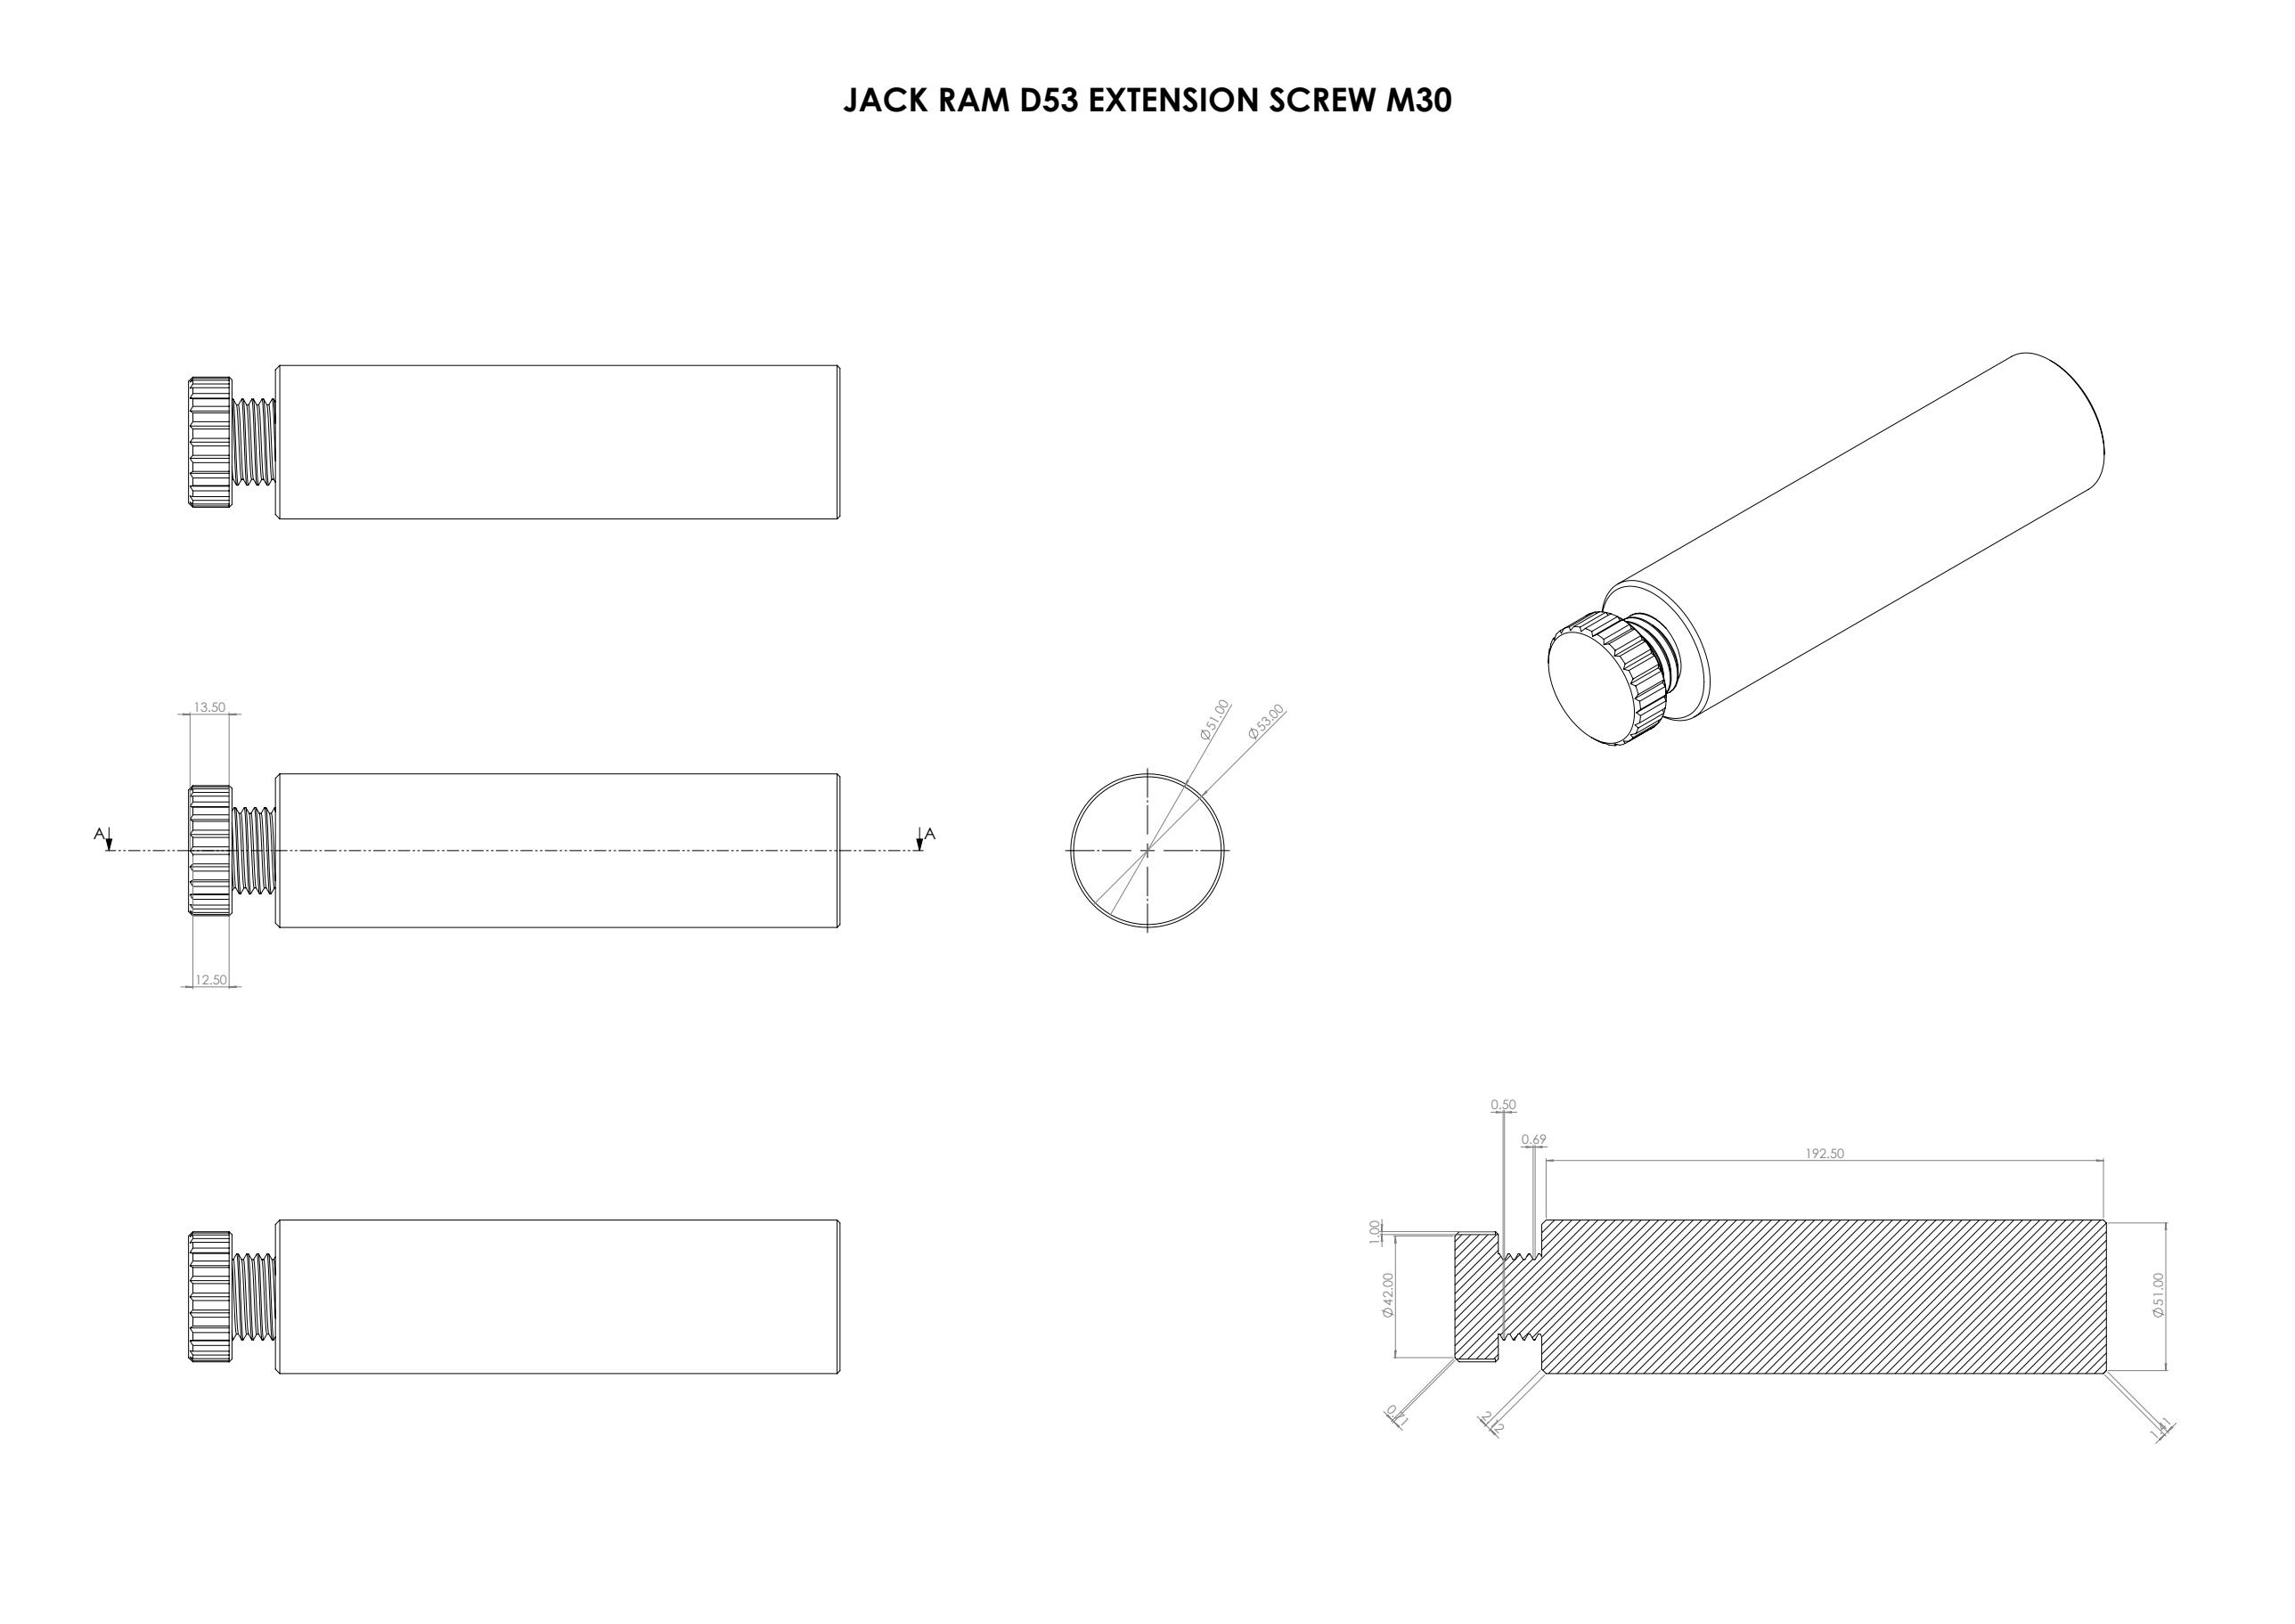
ISO-10303-21;
HEADER;
/* Generated by software containing ST-Developer
 * from STEP Tools, Inc. (www.steptools.com) 
 */

FILE_DESCRIPTION(
/* description */ (''),
/* implementation_level */ '2;1');

FILE_NAME(
/* name */ '10_Jack_Ram_D53_Extension_Screw_M30.step',
/* time_stamp */ '2026-10-20T10:03:03-07:00',
/* author */ (''),
/* organization */ (''),
/* preprocessor_version */ 'ST-DEVELOPER v20.2',
/* originating_system */ 'Autodesk Translation Framework v15.15.0.0',
/* authorisation */ '');

FILE_SCHEMA (('AUTOMOTIVE_DESIGN { 1 0 10303 214 3 1 1 }'));
ENDSEC;

DATA;
#10=MECHANICAL_DESIGN_GEOMETRIC_PRESENTATION_REPRESENTATION('',(#529),#71492);
#271=(
BOUNDED_CURVE()
B_SPLINE_CURVE(2,(#44561,#44562,#44563),.UNSPECIFIED.,.F.,.F.)
B_SPLINE_CURVE_WITH_KNOTS((3,3),(0.,0.186897942309885),.UNSPECIFIED.)
CURVE()
GEOMETRIC_REPRESENTATION_ITEM()
RATIONAL_B_SPLINE_CURVE((1.,1.00104922243968,1.00074449035823))
REPRESENTATION_ITEM('')
);
#272=(
BOUNDED_CURVE()
B_SPLINE_CURVE(2,(#44566,#44567,#44568),.UNSPECIFIED.,.F.,.F.)
B_SPLINE_CURVE_WITH_KNOTS((3,3),(0.102768382432289,0.289666324741965),
 .UNSPECIFIED.)
CURVE()
GEOMETRIC_REPRESENTATION_ITEM()
RATIONAL_B_SPLINE_CURVE((1.00074449035274,1.00104922243194,1.))
REPRESENTATION_ITEM('')
);
#273=(
BOUNDED_CURVE()
B_SPLINE_CURVE(2,(#44582,#44583,#44584),.UNSPECIFIED.,.F.,.F.)
B_SPLINE_CURVE_WITH_KNOTS((3,3),(0.,0.186897942309674),.UNSPECIFIED.)
CURVE()
GEOMETRIC_REPRESENTATION_ITEM()
RATIONAL_B_SPLINE_CURVE((1.,1.00104922243196,1.00074449035276))
REPRESENTATION_ITEM('')
);
#274=(
BOUNDED_CURVE()
B_SPLINE_CURVE(2,(#44587,#44588,#44589),.UNSPECIFIED.,.F.,.F.)
B_SPLINE_CURVE_WITH_KNOTS((3,3),(0.102768382432294,0.289666324741965),
 .UNSPECIFIED.)
CURVE()
GEOMETRIC_REPRESENTATION_ITEM()
RATIONAL_B_SPLINE_CURVE((1.00074449035267,1.00104922243184,1.))
REPRESENTATION_ITEM('')
);
#275=(
BOUNDED_CURVE()
B_SPLINE_CURVE(2,(#44603,#44604,#44605),.UNSPECIFIED.,.F.,.F.)
B_SPLINE_CURVE_WITH_KNOTS((3,3),(0.,0.186897942309901),.UNSPECIFIED.)
CURVE()
GEOMETRIC_REPRESENTATION_ITEM()
RATIONAL_B_SPLINE_CURVE((1.,1.00104922243998,1.00074449035845))
REPRESENTATION_ITEM('')
);
#276=(
BOUNDED_CURVE()
B_SPLINE_CURVE(2,(#44608,#44609,#44610),.UNSPECIFIED.,.F.,.F.)
B_SPLINE_CURVE_WITH_KNOTS((3,3),(0.102768382432298,0.289666324741965),
 .UNSPECIFIED.)
CURVE()
GEOMETRIC_REPRESENTATION_ITEM()
RATIONAL_B_SPLINE_CURVE((1.00074449035256,1.00104922243169,1.))
REPRESENTATION_ITEM('')
);
#277=(
BOUNDED_CURVE()
B_SPLINE_CURVE(2,(#44624,#44625,#44626),.UNSPECIFIED.,.F.,.F.)
B_SPLINE_CURVE_WITH_KNOTS((3,3),(0.,0.186897942309885),.UNSPECIFIED.)
CURVE()
GEOMETRIC_REPRESENTATION_ITEM()
RATIONAL_B_SPLINE_CURVE((1.,1.00104922243968,1.00074449035823))
REPRESENTATION_ITEM('')
);
#278=(
BOUNDED_CURVE()
B_SPLINE_CURVE(2,(#44629,#44630,#44631),.UNSPECIFIED.,.F.,.F.)
B_SPLINE_CURVE_WITH_KNOTS((3,3),(0.102768382432289,0.289666324741965),
 .UNSPECIFIED.)
CURVE()
GEOMETRIC_REPRESENTATION_ITEM()
RATIONAL_B_SPLINE_CURVE((1.00074449035274,1.00104922243194,1.))
REPRESENTATION_ITEM('')
);
#279=(
BOUNDED_CURVE()
B_SPLINE_CURVE(2,(#44645,#44646,#44647),.UNSPECIFIED.,.F.,.F.)
B_SPLINE_CURVE_WITH_KNOTS((3,3),(0.,0.186897942309671),.UNSPECIFIED.)
CURVE()
GEOMETRIC_REPRESENTATION_ITEM()
RATIONAL_B_SPLINE_CURVE((1.,1.00104922243187,1.00074449035269))
REPRESENTATION_ITEM('')
);
#280=(
BOUNDED_CURVE()
B_SPLINE_CURVE(2,(#44650,#44651,#44652),.UNSPECIFIED.,.F.,.F.)
B_SPLINE_CURVE_WITH_KNOTS((3,3),(0.102768382432295,0.289666324741964),
 .UNSPECIFIED.)
CURVE()
GEOMETRIC_REPRESENTATION_ITEM()
RATIONAL_B_SPLINE_CURVE((1.00074449035266,1.00104922243182,1.))
REPRESENTATION_ITEM('')
);
#281=(
BOUNDED_CURVE()
B_SPLINE_CURVE(2,(#44666,#44667,#44668),.UNSPECIFIED.,.F.,.F.)
B_SPLINE_CURVE_WITH_KNOTS((3,3),(0.,0.186897942309672),.UNSPECIFIED.)
CURVE()
GEOMETRIC_REPRESENTATION_ITEM()
RATIONAL_B_SPLINE_CURVE((1.,1.00104922243174,1.0007444903526))
REPRESENTATION_ITEM('')
);
#282=(
BOUNDED_CURVE()
B_SPLINE_CURVE(2,(#44671,#44672,#44673),.UNSPECIFIED.,.F.,.F.)
B_SPLINE_CURVE_WITH_KNOTS((3,3),(0.102768382432307,0.289666324741965),
 .UNSPECIFIED.)
CURVE()
GEOMETRIC_REPRESENTATION_ITEM()
RATIONAL_B_SPLINE_CURVE((1.00074449035222,1.00104922243121,1.))
REPRESENTATION_ITEM('')
);
#283=(
BOUNDED_CURVE()
B_SPLINE_CURVE(2,(#44689,#44690,#44691),.UNSPECIFIED.,.F.,.F.)
B_SPLINE_CURVE_WITH_KNOTS((3,3),(0.,0.186897942309665),.UNSPECIFIED.)
CURVE()
GEOMETRIC_REPRESENTATION_ITEM()
RATIONAL_B_SPLINE_CURVE((1.,1.00104922243153,1.00074449035245))
REPRESENTATION_ITEM('')
);
#284=(
BOUNDED_CURVE()
B_SPLINE_CURVE(2,(#44694,#44695,#44696),.UNSPECIFIED.,.F.,.F.)
B_SPLINE_CURVE_WITH_KNOTS((3,3),(0.102768382432301,0.289666324741966),
 .UNSPECIFIED.)
CURVE()
GEOMETRIC_REPRESENTATION_ITEM()
RATIONAL_B_SPLINE_CURVE((1.00074449035228,1.00104922243129,1.))
REPRESENTATION_ITEM('')
);
#285=(
BOUNDED_CURVE()
B_SPLINE_CURVE(2,(#44710,#44711,#44712),.UNSPECIFIED.,.F.,.F.)
B_SPLINE_CURVE_WITH_KNOTS((3,3),(0.,0.18689794230967),.UNSPECIFIED.)
CURVE()
GEOMETRIC_REPRESENTATION_ITEM()
RATIONAL_B_SPLINE_CURVE((1.,1.00104922243168,1.00074449035256))
REPRESENTATION_ITEM('')
);
#286=(
BOUNDED_CURVE()
B_SPLINE_CURVE(2,(#44715,#44716,#44717),.UNSPECIFIED.,.F.,.F.)
B_SPLINE_CURVE_WITH_KNOTS((3,3),(0.10276838243214,0.289666324741965),
 .UNSPECIFIED.)
CURVE()
GEOMETRIC_REPRESENTATION_ITEM()
RATIONAL_B_SPLINE_CURVE((1.00074449035625,1.00104922243688,1.))
REPRESENTATION_ITEM('')
);
#287=(
BOUNDED_CURVE()
B_SPLINE_CURVE(2,(#44731,#44732,#44733),.UNSPECIFIED.,.F.,.F.)
B_SPLINE_CURVE_WITH_KNOTS((3,3),(0.,0.186897942309663),.UNSPECIFIED.)
CURVE()
GEOMETRIC_REPRESENTATION_ITEM()
RATIONAL_B_SPLINE_CURVE((1.,1.00104922243133,1.00074449035231))
REPRESENTATION_ITEM('')
);
#288=(
BOUNDED_CURVE()
B_SPLINE_CURVE(2,(#44736,#44737,#44738),.UNSPECIFIED.,.F.,.F.)
B_SPLINE_CURVE_WITH_KNOTS((3,3),(0.102768382432299,0.289666324741965),
 .UNSPECIFIED.)
CURVE()
GEOMETRIC_REPRESENTATION_ITEM()
RATIONAL_B_SPLINE_CURVE((1.00074449035251,1.00104922243162,1.))
REPRESENTATION_ITEM('')
);
#289=(
BOUNDED_CURVE()
B_SPLINE_CURVE(2,(#44752,#44753,#44754),.UNSPECIFIED.,.F.,.F.)
B_SPLINE_CURVE_WITH_KNOTS((3,3),(0.,0.186897942309671),.UNSPECIFIED.)
CURVE()
GEOMETRIC_REPRESENTATION_ITEM()
RATIONAL_B_SPLINE_CURVE((1.,1.00104922243163,1.00074449035252))
REPRESENTATION_ITEM('')
);
#290=(
BOUNDED_CURVE()
B_SPLINE_CURVE(2,(#44757,#44758,#44759),.UNSPECIFIED.,.F.,.F.)
B_SPLINE_CURVE_WITH_KNOTS((3,3),(0.102768382432291,0.289666324741964),
 .UNSPECIFIED.)
CURVE()
GEOMETRIC_REPRESENTATION_ITEM()
RATIONAL_B_SPLINE_CURVE((1.00074449035272,1.00104922243191,1.))
REPRESENTATION_ITEM('')
);
#291=(
BOUNDED_CURVE()
B_SPLINE_CURVE(2,(#44773,#44774,#44775),.UNSPECIFIED.,.F.,.F.)
B_SPLINE_CURVE_WITH_KNOTS((3,3),(0.,0.186897942309668),.UNSPECIFIED.)
CURVE()
GEOMETRIC_REPRESENTATION_ITEM()
RATIONAL_B_SPLINE_CURVE((1.,1.00104922243145,1.00074449035239))
REPRESENTATION_ITEM('')
);
#292=(
BOUNDED_CURVE()
B_SPLINE_CURVE(2,(#44778,#44779,#44780),.UNSPECIFIED.,.F.,.F.)
B_SPLINE_CURVE_WITH_KNOTS((3,3),(0.102768382432079,0.289666324741965),
 .UNSPECIFIED.)
CURVE()
GEOMETRIC_REPRESENTATION_ITEM()
RATIONAL_B_SPLINE_CURVE((1.00074449035827,1.00104922243974,1.))
REPRESENTATION_ITEM('')
);
#293=(
BOUNDED_CURVE()
B_SPLINE_CURVE(2,(#44794,#44795,#44796),.UNSPECIFIED.,.F.,.F.)
B_SPLINE_CURVE_WITH_KNOTS((3,3),(0.,0.186897942309668),.UNSPECIFIED.)
CURVE()
GEOMETRIC_REPRESENTATION_ITEM()
RATIONAL_B_SPLINE_CURVE((1.,1.00104922243171,1.00074449035258))
REPRESENTATION_ITEM('')
);
#294=(
BOUNDED_CURVE()
B_SPLINE_CURVE(2,(#44799,#44800,#44801),.UNSPECIFIED.,.F.,.F.)
B_SPLINE_CURVE_WITH_KNOTS((3,3),(0.102768382432086,0.289666324741965),
 .UNSPECIFIED.)
CURVE()
GEOMETRIC_REPRESENTATION_ITEM()
RATIONAL_B_SPLINE_CURVE((1.00074449035837,1.00104922243988,1.))
REPRESENTATION_ITEM('')
);
#295=(
BOUNDED_CURVE()
B_SPLINE_CURVE(2,(#44815,#44816,#44817),.UNSPECIFIED.,.F.,.F.)
B_SPLINE_CURVE_WITH_KNOTS((3,3),(0.,0.186897942309671),.UNSPECIFIED.)
CURVE()
GEOMETRIC_REPRESENTATION_ITEM()
RATIONAL_B_SPLINE_CURVE((1.,1.00104922243187,1.00074449035269))
REPRESENTATION_ITEM('')
);
#296=(
BOUNDED_CURVE()
B_SPLINE_CURVE(2,(#44820,#44821,#44822),.UNSPECIFIED.,.F.,.F.)
B_SPLINE_CURVE_WITH_KNOTS((3,3),(0.102768382432293,0.289666324741965),
 .UNSPECIFIED.)
CURVE()
GEOMETRIC_REPRESENTATION_ITEM()
RATIONAL_B_SPLINE_CURVE((1.0007444903527,1.00104922243188,1.))
REPRESENTATION_ITEM('')
);
#297=(
BOUNDED_CURVE()
B_SPLINE_CURVE(2,(#44836,#44837,#44838),.UNSPECIFIED.,.F.,.F.)
B_SPLINE_CURVE_WITH_KNOTS((3,3),(0.,0.186897942309669),.UNSPECIFIED.)
CURVE()
GEOMETRIC_REPRESENTATION_ITEM()
RATIONAL_B_SPLINE_CURVE((1.,1.00104922243157,1.00074449035248))
REPRESENTATION_ITEM('')
);
#298=(
BOUNDED_CURVE()
B_SPLINE_CURVE(2,(#44841,#44842,#44843),.UNSPECIFIED.,.F.,.F.)
B_SPLINE_CURVE_WITH_KNOTS((3,3),(0.102768382432292,0.289666324741965),
 .UNSPECIFIED.)
CURVE()
GEOMETRIC_REPRESENTATION_ITEM()
RATIONAL_B_SPLINE_CURVE((1.00074449035271,1.00104922243189,1.))
REPRESENTATION_ITEM('')
);
#299=(
BOUNDED_CURVE()
B_SPLINE_CURVE(2,(#44857,#44858,#44859),.UNSPECIFIED.,.F.,.F.)
B_SPLINE_CURVE_WITH_KNOTS((3,3),(0.,0.186897942309658),.UNSPECIFIED.)
CURVE()
GEOMETRIC_REPRESENTATION_ITEM()
RATIONAL_B_SPLINE_CURVE((1.,1.00104922243123,1.00074449035224))
REPRESENTATION_ITEM('')
);
#300=(
BOUNDED_CURVE()
B_SPLINE_CURVE(2,(#44862,#44863,#44864),.UNSPECIFIED.,.F.,.F.)
B_SPLINE_CURVE_WITH_KNOTS((3,3),(0.102768382432307,0.289666324741965),
 .UNSPECIFIED.)
CURVE()
GEOMETRIC_REPRESENTATION_ITEM()
RATIONAL_B_SPLINE_CURVE((1.00074449035222,1.00104922243121,1.))
REPRESENTATION_ITEM('')
);
#301=(
BOUNDED_CURVE()
B_SPLINE_CURVE(2,(#44878,#44879,#44880),.UNSPECIFIED.,.F.,.F.)
B_SPLINE_CURVE_WITH_KNOTS((3,3),(0.,0.186897942309668),.UNSPECIFIED.)
CURVE()
GEOMETRIC_REPRESENTATION_ITEM()
RATIONAL_B_SPLINE_CURVE((1.,1.00104922243153,1.00074449035245))
REPRESENTATION_ITEM('')
);
#302=(
BOUNDED_CURVE()
B_SPLINE_CURVE(2,(#44883,#44884,#44885),.UNSPECIFIED.,.F.,.F.)
B_SPLINE_CURVE_WITH_KNOTS((3,3),(0.102768382432315,0.289666324741965),
 .UNSPECIFIED.)
CURVE()
GEOMETRIC_REPRESENTATION_ITEM()
RATIONAL_B_SPLINE_CURVE((1.00074449035217,1.00104922243113,1.))
REPRESENTATION_ITEM('')
);
#303=(
BOUNDED_CURVE()
B_SPLINE_CURVE(2,(#44899,#44900,#44901),.UNSPECIFIED.,.F.,.F.)
B_SPLINE_CURVE_WITH_KNOTS((3,3),(0.,0.186897942309684),.UNSPECIFIED.)
CURVE()
GEOMETRIC_REPRESENTATION_ITEM()
RATIONAL_B_SPLINE_CURVE((1.,1.00104922243195,1.00074449035275))
REPRESENTATION_ITEM('')
);
#304=(
BOUNDED_CURVE()
B_SPLINE_CURVE(2,(#44904,#44905,#44906),.UNSPECIFIED.,.F.,.F.)
B_SPLINE_CURVE_WITH_KNOTS((3,3),(0.102768382432288,0.289666324741966),
 .UNSPECIFIED.)
CURVE()
GEOMETRIC_REPRESENTATION_ITEM()
RATIONAL_B_SPLINE_CURVE((1.00074449035274,1.00104922243194,1.))
REPRESENTATION_ITEM('')
);
#305=(
BOUNDED_CURVE()
B_SPLINE_CURVE(2,(#44920,#44921,#44922),.UNSPECIFIED.,.F.,.F.)
B_SPLINE_CURVE_WITH_KNOTS((3,3),(0.,0.186897942309664),.UNSPECIFIED.)
CURVE()
GEOMETRIC_REPRESENTATION_ITEM()
RATIONAL_B_SPLINE_CURVE((1.,1.00104922243129,1.00074449035228))
REPRESENTATION_ITEM('')
);
#306=(
BOUNDED_CURVE()
B_SPLINE_CURVE(2,(#44925,#44926,#44927),.UNSPECIFIED.,.F.,.F.)
B_SPLINE_CURVE_WITH_KNOTS((3,3),(0.102768382432294,0.289666324741965),
 .UNSPECIFIED.)
CURVE()
GEOMETRIC_REPRESENTATION_ITEM()
RATIONAL_B_SPLINE_CURVE((1.00074449035262,1.00104922243177,1.))
REPRESENTATION_ITEM('')
);
#307=(
BOUNDED_CURVE()
B_SPLINE_CURVE(2,(#44941,#44942,#44943),.UNSPECIFIED.,.F.,.F.)
B_SPLINE_CURVE_WITH_KNOTS((3,3),(0.,0.186897942309668),.UNSPECIFIED.)
CURVE()
GEOMETRIC_REPRESENTATION_ITEM()
RATIONAL_B_SPLINE_CURVE((1.,1.00104922243147,1.00074449035241))
REPRESENTATION_ITEM('')
);
#308=(
BOUNDED_CURVE()
B_SPLINE_CURVE(2,(#44946,#44947,#44948),.UNSPECIFIED.,.F.,.F.)
B_SPLINE_CURVE_WITH_KNOTS((3,3),(0.102768382432086,0.289666324741965),
 .UNSPECIFIED.)
CURVE()
GEOMETRIC_REPRESENTATION_ITEM()
RATIONAL_B_SPLINE_CURVE((1.00074449035837,1.00104922243988,1.))
REPRESENTATION_ITEM('')
);
#309=(
BOUNDED_CURVE()
B_SPLINE_CURVE(2,(#44962,#44963,#44964),.UNSPECIFIED.,.F.,.F.)
B_SPLINE_CURVE_WITH_KNOTS((3,3),(0.,0.186897942309669),.UNSPECIFIED.)
CURVE()
GEOMETRIC_REPRESENTATION_ITEM()
RATIONAL_B_SPLINE_CURVE((1.,1.00104922243168,1.00074449035256))
REPRESENTATION_ITEM('')
);
#310=(
BOUNDED_CURVE()
B_SPLINE_CURVE(2,(#44967,#44968,#44969),.UNSPECIFIED.,.F.,.F.)
B_SPLINE_CURVE_WITH_KNOTS((3,3),(0.102768382432305,0.289666324741966),
 .UNSPECIFIED.)
CURVE()
GEOMETRIC_REPRESENTATION_ITEM()
RATIONAL_B_SPLINE_CURVE((1.0007444903522,1.00104922243117,1.))
REPRESENTATION_ITEM('')
);
#311=(
BOUNDED_CURVE()
B_SPLINE_CURVE(2,(#44983,#44984,#44985),.UNSPECIFIED.,.F.,.F.)
B_SPLINE_CURVE_WITH_KNOTS((3,3),(0.,0.186897942309671),.UNSPECIFIED.)
CURVE()
GEOMETRIC_REPRESENTATION_ITEM()
RATIONAL_B_SPLINE_CURVE((1.,1.00104922243178,1.00074449035262))
REPRESENTATION_ITEM('')
);
#312=(
BOUNDED_CURVE()
B_SPLINE_CURVE(2,(#44988,#44989,#44990),.UNSPECIFIED.,.F.,.F.)
B_SPLINE_CURVE_WITH_KNOTS((3,3),(0.102768382432293,0.289666324741965),
 .UNSPECIFIED.)
CURVE()
GEOMETRIC_REPRESENTATION_ITEM()
RATIONAL_B_SPLINE_CURVE((1.00074449035232,1.00104922243135,1.))
REPRESENTATION_ITEM('')
);
#313=(
BOUNDED_CURVE()
B_SPLINE_CURVE(2,(#45004,#45005,#45006),.UNSPECIFIED.,.F.,.F.)
B_SPLINE_CURVE_WITH_KNOTS((3,3),(0.,0.186897942309666),.UNSPECIFIED.)
CURVE()
GEOMETRIC_REPRESENTATION_ITEM()
RATIONAL_B_SPLINE_CURVE((1.,1.00104922243158,1.00074449035248))
REPRESENTATION_ITEM('')
);
#314=(
BOUNDED_CURVE()
B_SPLINE_CURVE(2,(#45009,#45010,#45011),.UNSPECIFIED.,.F.,.F.)
B_SPLINE_CURVE_WITH_KNOTS((3,3),(0.102768382432303,0.289666324741966),
 .UNSPECIFIED.)
CURVE()
GEOMETRIC_REPRESENTATION_ITEM()
RATIONAL_B_SPLINE_CURVE((1.00074449035238,1.00104922243143,1.))
REPRESENTATION_ITEM('')
);
#315=(
BOUNDED_CURVE()
B_SPLINE_CURVE(2,(#45025,#45026,#45027),.UNSPECIFIED.,.F.,.F.)
B_SPLINE_CURVE_WITH_KNOTS((3,3),(0.,0.186897942309666),.UNSPECIFIED.)
CURVE()
GEOMETRIC_REPRESENTATION_ITEM()
RATIONAL_B_SPLINE_CURVE((1.,1.00104922243159,1.00074449035249))
REPRESENTATION_ITEM('')
);
#316=(
BOUNDED_CURVE()
B_SPLINE_CURVE(2,(#45030,#45031,#45032),.UNSPECIFIED.,.F.,.F.)
B_SPLINE_CURVE_WITH_KNOTS((3,3),(0.102768382432302,0.289666324741967),
 .UNSPECIFIED.)
CURVE()
GEOMETRIC_REPRESENTATION_ITEM()
RATIONAL_B_SPLINE_CURVE((1.00074449035229,1.0010492224313,1.))
REPRESENTATION_ITEM('')
);
#317=(
BOUNDED_CURVE()
B_SPLINE_CURVE(2,(#45046,#45047,#45048),.UNSPECIFIED.,.F.,.F.)
B_SPLINE_CURVE_WITH_KNOTS((3,3),(0.,0.186897942309671),.UNSPECIFIED.)
CURVE()
GEOMETRIC_REPRESENTATION_ITEM()
RATIONAL_B_SPLINE_CURVE((1.,1.00104922243168,1.00074449035256))
REPRESENTATION_ITEM('')
);
#318=(
BOUNDED_CURVE()
B_SPLINE_CURVE(2,(#45051,#45052,#45053),.UNSPECIFIED.,.F.,.F.)
B_SPLINE_CURVE_WITH_KNOTS((3,3),(0.102768382432289,0.289666324741963),
 .UNSPECIFIED.)
CURVE()
GEOMETRIC_REPRESENTATION_ITEM()
RATIONAL_B_SPLINE_CURVE((1.00074449035275,1.00104922243195,1.))
REPRESENTATION_ITEM('')
);
#387=SHAPE_REPRESENTATION_RELATIONSHIP('SRR','None',#71608,#406);
#406=ADVANCED_BREP_SHAPE_REPRESENTATION('',(#425),#71478);
#425=MANIFOLD_SOLID_BREP('Ram',#28464);
#529=STYLED_ITEM('',(#71894),#425);
#785=B_SPLINE_CURVE_WITH_KNOTS('',3,(#44024,#44025,#44026,#44027,#44028,
#44029,#44030,#44031,#44032,#44033,#44034,#44035,#44036,#44037,#44038,#44039),
 .UNSPECIFIED.,.F.,.F.,(4,3,3,3,3,4),(-4.09305997722772,-3.86695282144916,
-3.38358371876801,-2.90021461608687,-2.41684551340572,-2.07420913009921),
 .UNSPECIFIED.);
#786=B_SPLINE_CURVE_WITH_KNOTS('',3,(#44042,#44043,#44044,#44045,#44046,
#44047,#44048,#44049,#44050,#44051),.UNSPECIFIED.,.F.,.F.,(4,3,3,4),(0.,
0.483369102681141,0.966738205362282,1.12274180646098),.UNSPECIFIED.);
#787=B_SPLINE_CURVE_WITH_KNOTS('',3,(#44056,#44057,#44058,#44059,#44060,
#44061,#44062,#44063,#44064,#44065,#44066,#44067,#44068,#44069,#44070,#44071,
#44072,#44073,#44074,#44075,#44076,#44077,#44078,#44079,#44080,#44081,#44082,
#44083,#44084,#44085,#44086,#44087,#44088,#44089,#44090,#44091,#44092,#44093,
#44094,#44095,#44096,#44097,#44098),.UNSPECIFIED.,.F.,.F.,(4,3,3,3,3,3,
3,3,3,3,3,3,3,3,4),(-10.3762452844077,-10.150751156304,-9.6673820536229,
-9.18401295094176,-8.70064384826061,-8.21727474557946,-7.73390564289832,
-7.25053654021717,-6.76716743753603,-6.28379833485489,-5.80042923217374,
-5.3170601294926,-4.83369102681145,-4.35032192413031,-4.09305997722772),
 .UNSPECIFIED.);
#788=B_SPLINE_CURVE_WITH_KNOTS('',3,(#44099,#44100,#44101,#44102,#44103,
#44104,#44105,#44106,#44107,#44108,#44109,#44110,#44111,#44112,#44113,#44114,
#44115,#44116,#44117,#44118,#44119,#44120,#44121,#44122,#44123,#44124,#44125,
#44126,#44127,#44128,#44129,#44130,#44131,#44132,#44133,#44134,#44135,#44136,
#44137,#44138,#44139,#44140,#44141),.UNSPECIFIED.,.F.,.F.,(4,3,3,3,3,3,
3,3,3,3,3,3,3,3,4),(1.12274180646098,1.45010730804342,1.93347641072457,
2.41684551340571,2.90021461608685,3.38358371876799,3.86695282144913,4.35032192413027,
4.83369102681141,5.31706012949256,5.8004292321737,6.28379833485484,6.76716743753598,
7.25053654021712,7.40592711364047),.UNSPECIFIED.);
#789=B_SPLINE_CURVE_WITH_KNOTS('',3,(#44146,#44147,#44148,#44149,#44150,
#44151,#44152,#44153,#44154,#44155,#44156,#44157,#44158,#44159,#44160,#44161,
#44162,#44163,#44164,#44165,#44166,#44167,#44168,#44169,#44170,#44171,#44172,
#44173,#44174,#44175,#44176,#44177,#44178,#44179,#44180,#44181,#44182,#44183,
#44184,#44185,#44186,#44187,#44188),.UNSPECIFIED.,.F.,.F.,(4,3,3,3,3,3,
3,3,3,3,3,3,3,3,4),(-16.6594305915872,-16.4345494911589,-15.9511803884778,
-15.4678112857966,-14.9844421831155,-14.5010730804343,-14.0177039777532,
-13.5343348750721,-13.0509657723909,-12.5675966697098,-12.0842275670286,
-11.6008584643475,-11.1174893616663,-10.6341202589852,-10.3762452844077),
 .UNSPECIFIED.);
#790=B_SPLINE_CURVE_WITH_KNOTS('',3,(#44189,#44190,#44191,#44192,#44193,
#44194,#44195,#44196,#44197,#44198,#44199,#44200,#44201,#44202,#44203,#44204,
#44205,#44206,#44207,#44208,#44209,#44210,#44211,#44212,#44213,#44214,#44215,
#44216,#44217,#44218,#44219,#44220,#44221,#44222,#44223,#44224,#44225,#44226,
#44227,#44228,#44229,#44230,#44231),.UNSPECIFIED.,.F.,.F.,(4,3,3,3,3,3,
3,3,3,3,3,3,3,3,4),(7.40592711364047,7.73390564289826,8.2172747455794,8.70064384826054,
9.18401295094169,9.66738205362283,10.150751156304,10.6341202589851,11.1174893616663,
11.6008584643474,12.0842275670285,12.5675966697097,13.0509657723908,13.534334875072,
13.6891124208199),.UNSPECIFIED.);
#791=B_SPLINE_CURVE_WITH_KNOTS('',3,(#44236,#44237,#44238,#44239,#44240,
#44241,#44242,#44243,#44244,#44245,#44246,#44247,#44248,#44249,#44250,#44251,
#44252,#44253,#44254,#44255,#44256,#44257,#44258,#44259,#44260,#44261,#44262,
#44263,#44264,#44265,#44266,#44267,#44268,#44269,#44270,#44271,#44272,#44273,
#44274,#44275,#44276,#44277,#44278),.UNSPECIFIED.,.F.,.F.,(4,3,3,3,3,3,
3,3,3,3,3,3,3,3,4),(-22.9426158987667,-22.7183478260138,-22.2349787233327,
-21.7516096206515,-21.2682405179704,-20.7848714152892,-20.3015023126081,
-19.8181332099269,-19.3347641072458,-18.8513950045647,-18.3680259018835,
-17.8846567992024,-17.4012876965212,-16.9179185938401,-16.6594305915872),
 .UNSPECIFIED.);
#792=B_SPLINE_CURVE_WITH_KNOTS('',3,(#44279,#44280,#44281,#44282,#44283,
#44284,#44285,#44286,#44287,#44288,#44289,#44290,#44291,#44292,#44293,#44294,
#44295,#44296,#44297,#44298,#44299,#44300,#44301,#44302,#44303,#44304,#44305,
#44306,#44307,#44308,#44309,#44310,#44311,#44312,#44313,#44314,#44315,#44316,
#44317,#44318,#44319,#44320,#44321),.UNSPECIFIED.,.F.,.F.,(4,3,3,3,3,3,
3,3,3,3,3,3,3,3,4),(13.6891124208199,14.0177039777531,14.5010730804342,
14.9844421831154,15.4678112857965,15.9511803884777,16.4345494911588,16.9179185938399,
17.4012876965211,17.8846567992022,18.3680259018834,18.8513950045645,19.3347641072457,
19.8181332099268,19.9722977279999),.UNSPECIFIED.);
#793=B_SPLINE_CURVE_WITH_KNOTS('',3,(#44328,#44329,#44330,#44331,#44332,
#44333,#44334,#44335,#44336,#44337,#44338,#44339,#44340,#44341,#44342,#44343,
#44344,#44345,#44346,#44347,#44348,#44349,#44350,#44351,#44352,#44353,#44354,
#44355,#44356,#44357,#44358,#44359,#44360,#44361,#44362,#44363,#44364,#44365,
#44366,#44367),.UNSPECIFIED.,.F.,.F.,(4,3,3,3,3,3,3,3,3,3,3,3,3,4),(-29.0021461608684,
-28.5187770581875,-28.0354079555064,-27.5520388528253,-27.0686697501441,
-26.585300647463,-26.1019315447818,-25.6185624421007,-25.1351933394195,
-24.6518242367384,-24.1684551340572,-23.6850860313761,-23.201716928695,
-22.9426158987667),.UNSPECIFIED.);
#794=B_SPLINE_CURVE_WITH_KNOTS('',3,(#44368,#44369,#44370,#44371,#44372,
#44373,#44374,#44375,#44376,#44377,#44378,#44379,#44380,#44381,#44382,#44383,
#44384,#44385,#44386,#44387,#44388,#44389,#44390,#44391,#44392,#44393,#44394,
#44395,#44396,#44397,#44398,#44399,#44400,#44401,#44402,#44403,#44404,#44405,
#44406,#44407,#44408,#44409,#44410),.UNSPECIFIED.,.F.,.F.,(4,3,3,3,3,3,
3,3,3,3,3,3,3,3,4),(19.9722977279999,20.3015023126079,20.7848714152891,
21.2682405179702,21.7516096206514,22.2349787233325,22.7183478260136,23.2017169286948,
23.6850860313759,24.1684551340571,24.6518242367382,25.1351933394193,25.6185624421005,
26.1019315447816,26.2554830351794),.UNSPECIFIED.);
#795=B_SPLINE_CURVE_WITH_KNOTS('',3,(#44416,#44417,#44418,#44419,#44420,
#44421,#44422,#44423,#44424,#44425,#44426,#44427),.UNSPECIFIED.,.F.,.F.,
(4,1,1,1,1,1,1,1,1,4),(34.5575191894879,34.816620219416,35.2999893220971,
35.7833584247782,36.2667275274594,36.7500966301405,37.2334657328217,37.7168348355028,
38.200203938184,38.5428403214904),.UNSPECIFIED.);
#796=B_SPLINE_CURVE_WITH_KNOTS('',3,(#44430,#44431,#44432,#44433,#44434,
#44435,#44436,#44437,#44438),.UNSPECIFIED.,.F.,.F.,(4,1,1,1,1,1,4),(34.5575191894879,
34.8873368017712,35.3707059044523,35.8540750071334,36.3374441098146,36.8208132124957,
37.3041823151769),.UNSPECIFIED.);
#797=B_SPLINE_CURVE_WITH_KNOTS('',3,(#44443,#44444,#44445,#44446,#44447,
#44448,#44449,#44450,#44451,#44452,#44453,#44454,#44455,#44456,#44457,#44458,
#44459),.UNSPECIFIED.,.F.,.F.,(4,1,1,1,1,1,1,1,1,1,1,1,1,1,4),(28.2743338823079,
28.5328218845611,29.0161909872422,29.4995600899234,29.9829291926045,30.4662982952857,
30.9496673979668,31.4330365006479,31.9164056033291,32.3997747060102,32.8831438086914,
33.3665129113725,33.8498820140537,34.3332511167348,34.5575191894879),
 .UNSPECIFIED.);
#798=B_SPLINE_CURVE_WITH_KNOTS('',3,(#44460,#44461,#44462,#44463,#44464,
#44465,#44466,#44467,#44468,#44469,#44470,#44471,#44472,#44473,#44474,#44475,
#44476),.UNSPECIFIED.,.F.,.F.,(4,1,1,1,1,1,1,1,1,1,1,1,1,1,4),(28.2743338823079,
28.6035384669163,29.0869075695975,29.5702766722786,30.0536457749597,30.5370148776409,
31.020383980322,31.5037530830032,31.9871221856843,32.4704912883655,32.9538603910466,
33.4372294937277,33.9205985964089,34.40396769909,34.5575191894879),
 .UNSPECIFIED.);
#799=B_SPLINE_CURVE_WITH_KNOTS('',3,(#44481,#44482,#44483,#44484,#44485,
#44486,#44487,#44488,#44489,#44490,#44491,#44492,#44493,#44494,#44495,#44496,
#44497),.UNSPECIFIED.,.F.,.F.,(4,1,1,1,1,1,1,1,1,1,1,1,1,1,4),(21.9911485751285,
22.2490235497062,22.7323926523873,23.2157617550685,23.6991308577496,24.1824999604308,
24.6658690631119,25.1492381657931,25.6326072684742,26.1159763711553,26.5993454738365,
27.0827145765176,27.5660836791988,28.0494527818799,28.2743338823079),
 .UNSPECIFIED.);
#800=B_SPLINE_CURVE_WITH_KNOTS('',3,(#44498,#44499,#44500,#44501,#44502,
#44503,#44504,#44505,#44506,#44507,#44508,#44509,#44510,#44511,#44512,#44513,
#44514),.UNSPECIFIED.,.F.,.F.,(4,1,1,1,1,1,1,1,1,1,1,1,1,1,4),(21.9911485751284,
22.3197401320615,22.8031092347426,23.2864783374238,23.7698474401049,24.253216542786,
24.7365856454672,25.2199547481483,25.7033238508295,26.1866929535106,26.6700620561917,
27.1534311588729,27.636800261554,28.1201693642352,28.2743338823079),
 .UNSPECIFIED.);
#801=B_SPLINE_CURVE_WITH_KNOTS('',3,(#44519,#44520,#44521,#44522,#44523,
#44524,#44525,#44526,#44527,#44528,#44529,#44530,#44531,#44532,#44533,#44534,
#44535),.UNSPECIFIED.,.F.,.F.,(4,1,1,1,1,1,1,1,1,1,1,1,1,1,4),(15.707963267949,
15.9652252148513,16.4485943175325,16.9319634202136,17.4153325228947,17.8987016255759,
18.382070728257,18.8654398309382,19.3488089336193,19.8321780363005,20.3155471389816,
20.7989162416628,21.2822853443439,21.765654447025,21.9911485751285),
 .UNSPECIFIED.);
#802=B_SPLINE_CURVE_WITH_KNOTS('',3,(#44536,#44537,#44538,#44539,#44540,
#44541,#44542,#44543,#44544,#44545,#44546,#44547,#44548,#44549,#44550,#44551,
#44552),.UNSPECIFIED.,.F.,.F.,(4,1,1,1,1,1,1,1,1,1,1,1,1,1,4),(15.707963267949,
16.0359417972066,16.5193108998878,17.0026800025689,17.4860491052501,17.9694182079312,
18.4527873106123,18.9361564132935,19.4195255159746,19.9028946186558,20.3862637213369,
20.8696328240181,21.3530019266992,21.8363710293803,21.9911485751284),
 .UNSPECIFIED.);
#803=B_SPLINE_CURVE_WITH_KNOTS('',3,(#45386,#45387,#45388,#45389,#45390,
#45391,#45392,#45393,#45394,#45395,#45396,#45397,#45398,#45399,#45400,#45401,
#45402,#45403,#45404,#45405,#45406,#45407,#45408,#45409,#45410,#45411,#45412,
#45413,#45414,#45415,#45416,#45417,#45418,#45419,#45420,#45421,#45422,#45423,
#45424,#45425,#45426,#45427,#45428,#45429,#45430,#45431,#45432,#45433,#45434,
#45435,#45436,#45437,#45438,#45439,#45440,#45441,#45442,#45443,#45444,#45445,
#45446,#45447,#45448,#45449,#45450,#45451,#45452,#45453,#45454,#45455,#45456,
#45457,#45458,#45459,#45460,#45461,#45462,#45463,#45464,#45465,#45466,#45467,
#45468,#45469,#45470,#45471,#45472,#45473,#45474,#45475,#45476),
 .UNSPECIFIED.,.F.,.F.,(4,3,3,3,3,3,3,3,3,3,3,3,3,3,3,3,3,3,3,3,3,3,3,3,
3,3,3,3,3,3,4),(-2.88655140298914,-2.7102193708046,-2.67807220368065,-2.55828267008941,
-2.50176083674511,-2.46325112464318,-2.28839166473607,-2.20291800933891,
-2.13297054348664,-2.09735834895935,-1.9763367136572,-1.80417085977603,
-1.67697657920847,-1.61936340605544,-1.58062902684361,-1.54800677498682,
-1.37969242088531,-1.29539373750579,-1.1306741467308,-1.06564221343476,
-1.03346927595282,-1.00237020411154,-0.837024911419402,-0.673735787434826,
-0.63651537440582,-0.556950952605093,-0.517031410677791,-0.487820375823624,
-0.32585266849659,-0.162926334248295,0.),.UNSPECIFIED.);
#804=B_SPLINE_CURVE_WITH_KNOTS('',3,(#45477,#45478,#45479,#45480,#45481,
#45482,#45483),.UNSPECIFIED.,.F.,.F.,(4,3,4),(26.2554830351794,26.5853006474628,
26.9279370307691),.UNSPECIFIED.);
#805=B_SPLINE_CURVE_WITH_KNOTS('',3,(#45485,#45486,#45487,#45488,#45489,
#45490,#45491,#45492,#45493,#45494,#45495,#45496,#45497,#45498,#45499,#45500,
#45501,#45502,#45503,#45504,#45505,#45506,#45507,#45508,#45509,#45510,#45511,
#45512,#45513,#45514,#45515,#45516,#45517,#45518,#45519,#45520,#45521,#45522,
#45523,#45524,#45525,#45526,#45527,#45528,#45529,#45530,#45531,#45532,#45533,
#45534,#45535,#45536,#45537,#45538,#45539,#45540,#45541,#45542,#45543,#45544,
#45545,#45546,#45547,#45548,#45549,#45550,#45551,#45552,#45553,#45554,#45555,
#45556,#45557,#45558,#45559,#45560,#45561,#45562,#45563,#45564,#45565,#45566,
#45567,#45568,#45569,#45570,#45571,#45572,#45573,#45574,#45575),
 .UNSPECIFIED.,.F.,.F.,(4,3,3,3,3,3,3,3,3,3,3,3,3,3,3,3,3,3,3,3,3,3,3,3,
3,3,3,3,3,3,4),(-2.89533449801215,-2.73352650875014,-2.71205820706862,-2.59373915178661,
-2.55473003463996,-2.51830819618893,-2.35467992623886,-2.26957883251844,
-2.22055522388971,-2.18083698788503,-2.06810318921435,-1.90126059971141,
-1.77612865758421,-1.71255672102284,-1.67447106332452,-1.64582559314776,
-1.47561435227979,-1.4007328312026,-1.22836140698568,-1.15826779788408,
-1.12728054073534,-0.955264412683464,-0.781353242222385,-0.711247134334915,
-0.62234124254305,-0.578011318404134,-0.547059489792038,-0.371624702645109,
-0.185812351322555,-0.0101929273281714,0.),.UNSPECIFIED.);
#806=B_SPLINE_CURVE_WITH_KNOTS('',3,(#45576,#45577,#45578,#45579,#45580,
#45581,#45582,#45583,#45584,#45585,#45586,#45587,#45588,#45589,#45590),
 .UNSPECIFIED.,.F.,.F.,(4,1,1,1,1,1,1,1,1,1,1,1,4),(10.3762452844077,10.7188816677141,
11.2022507703952,11.6856198730764,12.1689889757575,12.6523580784387,13.1357271811198,
13.6190962838009,14.1024653864821,14.5858344891632,15.0692035918444,15.5525726945255,
15.707963267949),.UNSPECIFIED.);
#807=B_SPLINE_CURVE_WITH_KNOTS('',3,(#45594,#45595,#45596,#45597,#45598,
#45599,#45600,#45601,#45602,#45603,#45604,#45605),.UNSPECIFIED.,.F.,.F.,
(4,1,1,1,1,1,1,1,1,4),(11.614903290721,12.0982723934021,12.5816414960833,
13.0650105987644,13.5483797014456,14.0317488041267,14.5151179068079,14.998487009489,
15.4818561121702,15.707963267949),.UNSPECIFIED.);
#808=B_SPLINE_CURVE_WITH_KNOTS('',3,(#45858,#45859,#45860,#45861,#45862,
#45863,#45864,#45865,#45866,#45867,#45868,#45869,#45870,#45871,#45872,#45873,
#45874,#45875,#45876,#45877,#45878,#45879,#45880,#45881,#45882,#45883,#45884,
#45885,#45886,#45887,#45888,#45889,#45890,#45891,#45892,#45893,#45894,#45895,
#45896,#45897,#45898,#45899,#45900,#45901,#45902,#45903,#45904,#45905,#45906,
#45907,#45908,#45909,#45910,#45911,#45912,#45913,#45914,#45915,#45916,#45917,
#45918,#45919,#45920,#45921,#45922,#45923,#45924,#45925,#45926,#45927,#45928,
#45929,#45930,#45931,#45932,#45933,#45934,#45935,#45936,#45937,#45938,#45939,
#45940,#45941,#45942,#45943,#45944,#45945,#45946,#45947,#45948),
 .UNSPECIFIED.,.F.,.F.,(4,3,3,3,3,3,3,3,3,3,3,3,3,3,3,3,3,3,3,3,3,3,3,3,
3,3,3,3,3,3,4),(-2.89533449801219,-2.73352650875626,-2.71205820706864,-2.59373915175461,
-2.55473003455109,-2.51830819619465,-2.35467992625535,-2.26957883246004,
-2.22055522381054,-2.1808369878803,-2.06810318921433,-1.90126059971139,
-1.77612865758419,-1.71255672104602,-1.67447106339855,-1.64582559316971,
-1.47561435224765,-1.40073283120257,-1.22836140698566,-1.15826779788333,
-1.12728054084049,-0.955264412620505,-0.781353242677817,-0.711247134334909,
-0.622341242543046,-0.578011318009217,-0.547059488903834,-0.371624703144557,
-0.185812351572279,-0.0101929249643171,0.),.UNSPECIFIED.);
#809=B_SPLINE_CURVE_WITH_KNOTS('',3,(#45949,#45950,#45951,#45952,#45953,
#45954,#45955,#45956,#45957,#45958,#45959,#45960,#45961,#45962,#45963,#45964,
#45965,#45966,#45967,#45968,#45969,#45970,#45971,#45972,#45973,#45974,#45975,
#45976,#45977,#45978,#45979,#45980,#45981,#45982,#45983,#45984,#45985,#45986,
#45987,#45988,#45989,#45990,#45991,#45992,#45993,#45994,#45995,#45996,#45997,
#45998,#45999,#46000,#46001,#46002,#46003,#46004,#46005,#46006,#46007,#46008,
#46009,#46010,#46011,#46012,#46013,#46014,#46015,#46016,#46017,#46018,#46019,
#46020,#46021,#46022,#46023,#46024,#46025,#46026,#46027,#46028,#46029,#46030,
#46031,#46032,#46033,#46034,#46035,#46036,#46037,#46038,#46039),
 .UNSPECIFIED.,.F.,.F.,(4,3,3,3,3,3,3,3,3,3,3,3,3,3,3,3,3,3,3,3,3,3,3,3,
3,3,3,3,3,3,4),(-2.8865514029894,-2.7102193707971,-2.67807220368071,-2.55828267024697,
-2.50176083711203,-2.46325112472949,-2.28839166475814,-2.20291800935664,
-2.13297054351986,-2.09735834899737,-1.97633671365723,-1.8041708597012,
-1.67697657915235,-1.61936340596183,-1.58062902659333,-1.54800677505344,
-1.37969242083436,-1.2953937375058,-1.13067414673081,-1.06564221343148,
-1.03346927589314,-1.00237020410157,-0.837024911918307,-0.67373578950061,
-0.636515374405833,-0.556950952605104,-0.517031410437666,-0.48782037559651,
-0.325852668022188,-0.162926334011094,0.),.UNSPECIFIED.);
#1454=B_SPLINE_SURFACE_WITH_KNOTS('',3,3,((#45133,#45134,#45135,#45136,
#45137,#45138,#45139,#45140,#45141,#45142,#45143,#45144,#45145,#45146,#45147,
#45148,#45149,#45150,#45151,#45152,#45153,#45154,#45155,#45156,#45157,#45158,
#45159,#45160,#45161,#45162,#45163,#45164,#45165,#45166,#45167,#45168,#45169,
#45170,#45171,#45172,#45173,#45174,#45175,#45176,#45177,#45178,#45179,#45180,
#45181,#45182,#45183,#45184,#45185,#45186,#45187,#45188,#45189,#45190,#45191,
#45192,#45193,#45194,#45195),(#45196,#45197,#45198,#45199,#45200,#45201,
#45202,#45203,#45204,#45205,#45206,#45207,#45208,#45209,#45210,#45211,#45212,
#45213,#45214,#45215,#45216,#45217,#45218,#45219,#45220,#45221,#45222,#45223,
#45224,#45225,#45226,#45227,#45228,#45229,#45230,#45231,#45232,#45233,#45234,
#45235,#45236,#45237,#45238,#45239,#45240,#45241,#45242,#45243,#45244,#45245,
#45246,#45247,#45248,#45249,#45250,#45251,#45252,#45253,#45254,#45255,#45256,
#45257,#45258),(#45259,#45260,#45261,#45262,#45263,#45264,#45265,#45266,
#45267,#45268,#45269,#45270,#45271,#45272,#45273,#45274,#45275,#45276,#45277,
#45278,#45279,#45280,#45281,#45282,#45283,#45284,#45285,#45286,#45287,#45288,
#45289,#45290,#45291,#45292,#45293,#45294,#45295,#45296,#45297,#45298,#45299,
#45300,#45301,#45302,#45303,#45304,#45305,#45306,#45307,#45308,#45309,#45310,
#45311,#45312,#45313,#45314,#45315,#45316,#45317,#45318,#45319,#45320,#45321),
(#45322,#45323,#45324,#45325,#45326,#45327,#45328,#45329,#45330,#45331,
#45332,#45333,#45334,#45335,#45336,#45337,#45338,#45339,#45340,#45341,#45342,
#45343,#45344,#45345,#45346,#45347,#45348,#45349,#45350,#45351,#45352,#45353,
#45354,#45355,#45356,#45357,#45358,#45359,#45360,#45361,#45362,#45363,#45364,
#45365,#45366,#45367,#45368,#45369,#45370,#45371,#45372,#45373,#45374,#45375,
#45376,#45377,#45378,#45379,#45380,#45381,#45382,#45383,#45384)),
 .UNSPECIFIED.,.F.,.F.,.F.,(4,4),(4,1,1,1,1,1,1,1,1,1,1,1,1,1,1,1,1,1,1,
1,1,1,1,1,1,1,1,1,1,1,1,1,1,1,1,1,1,1,1,1,1,1,1,1,1,1,1,1,1,1,1,1,1,1,1,
1,1,1,1,1,4),(0.,0.231084445243146),(8.30203615430838,8.78540525698952,
9.26877435967066,9.7521434623518,10.2355125650329,10.7188816677141,11.2022507703952,
11.6856198730764,12.1689889757575,12.6523580784387,13.1357271811198,13.6190962838009,
14.1024653864821,14.5858344891632,15.0692035918444,15.5525726945255,16.0359417972066,
16.5193108998878,17.0026800025689,17.4860491052501,17.9694182079312,18.4527873106123,
18.9361564132935,19.4195255159746,19.9028946186558,20.3862637213369,20.8696328240181,
21.3530019266992,21.8363710293803,22.3197401320615,22.8031092347426,23.2864783374238,
23.7698474401049,24.253216542786,24.7365856454672,25.2199547481483,25.7033238508295,
26.1866929535106,26.6700620561917,27.1534311588729,27.636800261554,28.1201693642352,
28.6035384669163,29.0869075695975,29.5702766722786,30.0536457749597,30.5370148776409,
31.020383980322,31.5037530830032,31.9871221856843,32.4704912883655,32.9538603910466,
33.4372294937277,33.9205985964089,34.40396769909,34.8873368017712,35.3707059044523,
35.8540750071334,36.3374441098146,36.8208132124957,37.3041823151769),
 .UNSPECIFIED.);
#1455=B_SPLINE_SURFACE_WITH_KNOTS('',3,3,((#45606,#45607,#45608,#45609,
#45610,#45611,#45612,#45613,#45614,#45615,#45616,#45617,#45618,#45619,#45620,
#45621,#45622,#45623,#45624,#45625,#45626,#45627,#45628,#45629,#45630,#45631,
#45632,#45633,#45634,#45635,#45636,#45637,#45638,#45639,#45640,#45641,#45642,
#45643,#45644,#45645,#45646,#45647,#45648,#45649,#45650,#45651,#45652,#45653,
#45654,#45655,#45656,#45657,#45658,#45659,#45660,#45661,#45662,#45663,#45664,
#45665,#45666,#45667,#45668),(#45669,#45670,#45671,#45672,#45673,#45674,
#45675,#45676,#45677,#45678,#45679,#45680,#45681,#45682,#45683,#45684,#45685,
#45686,#45687,#45688,#45689,#45690,#45691,#45692,#45693,#45694,#45695,#45696,
#45697,#45698,#45699,#45700,#45701,#45702,#45703,#45704,#45705,#45706,#45707,
#45708,#45709,#45710,#45711,#45712,#45713,#45714,#45715,#45716,#45717,#45718,
#45719,#45720,#45721,#45722,#45723,#45724,#45725,#45726,#45727,#45728,#45729,
#45730,#45731),(#45732,#45733,#45734,#45735,#45736,#45737,#45738,#45739,
#45740,#45741,#45742,#45743,#45744,#45745,#45746,#45747,#45748,#45749,#45750,
#45751,#45752,#45753,#45754,#45755,#45756,#45757,#45758,#45759,#45760,#45761,
#45762,#45763,#45764,#45765,#45766,#45767,#45768,#45769,#45770,#45771,#45772,
#45773,#45774,#45775,#45776,#45777,#45778,#45779,#45780,#45781,#45782,#45783,
#45784,#45785,#45786,#45787,#45788,#45789,#45790,#45791,#45792,#45793,#45794),
(#45795,#45796,#45797,#45798,#45799,#45800,#45801,#45802,#45803,#45804,
#45805,#45806,#45807,#45808,#45809,#45810,#45811,#45812,#45813,#45814,#45815,
#45816,#45817,#45818,#45819,#45820,#45821,#45822,#45823,#45824,#45825,#45826,
#45827,#45828,#45829,#45830,#45831,#45832,#45833,#45834,#45835,#45836,#45837,
#45838,#45839,#45840,#45841,#45842,#45843,#45844,#45845,#45846,#45847,#45848,
#45849,#45850,#45851,#45852,#45853,#45854,#45855,#45856,#45857)),
 .UNSPECIFIED.,.F.,.F.,.F.,(4,4),(4,1,1,1,1,1,1,1,1,1,1,1,1,1,1,1,1,1,1,
1,1,1,1,1,1,1,1,1,1,1,1,1,1,1,1,1,1,1,1,1,1,1,1,1,1,1,1,1,1,1,1,1,1,1,1,
1,1,1,1,1,4),(0.,0.231084445243146),(11.614903290721,12.0982723934021,12.5816414960833,
13.0650105987644,13.5483797014456,14.0317488041267,14.5151179068079,14.998487009489,
15.4818561121702,15.9652252148513,16.4485943175325,16.9319634202136,17.4153325228947,
17.8987016255759,18.382070728257,18.8654398309382,19.3488089336193,19.8321780363005,
20.3155471389816,20.7989162416628,21.2822853443439,21.765654447025,22.2490235497062,
22.7323926523873,23.2157617550685,23.6991308577496,24.1824999604308,24.6658690631119,
25.1492381657931,25.6326072684742,26.1159763711553,26.5993454738365,27.0827145765176,
27.5660836791988,28.0494527818799,28.5328218845611,29.0161909872422,29.4995600899234,
29.9829291926045,30.4662982952857,30.9496673979668,31.4330365006479,31.9164056033291,
32.3997747060102,32.8831438086914,33.3665129113725,33.8498820140537,34.3332511167348,
34.816620219416,35.2999893220971,35.7833584247782,36.2667275274594,36.7500966301405,
37.2334657328217,37.7168348355028,38.200203938184,38.6835730408651,39.1669421435463,
39.6503112462274,40.1336803489085,40.6170494515897),.UNSPECIFIED.);
#1592=CYLINDRICAL_SURFACE('',#29536,1.486725);
#1593=CYLINDRICAL_SURFACE('',#29538,1.486725);
#1594=CYLINDRICAL_SURFACE('',#29539,1.486725);
#1595=CYLINDRICAL_SURFACE('',#29540,1.486725);
#1596=CYLINDRICAL_SURFACE('',#29541,1.486725);
#1597=CYLINDRICAL_SURFACE('',#29543,1.2866);
#1598=CYLINDRICAL_SURFACE('',#29545,1.2866);
#1599=CYLINDRICAL_SURFACE('',#29546,1.2866);
#1600=CYLINDRICAL_SURFACE('',#29547,1.2866);
#1601=CYLINDRICAL_SURFACE('',#29671,2.25);
#1602=CYLINDRICAL_SURFACE('',#29673,2.25);
#1603=CYLINDRICAL_SURFACE('',#29675,2.25);
#1604=CYLINDRICAL_SURFACE('',#29677,2.25);
#1605=CYLINDRICAL_SURFACE('',#29679,2.25);
#1606=CYLINDRICAL_SURFACE('',#29681,2.25);
#1607=CYLINDRICAL_SURFACE('',#29683,2.25);
#1608=CYLINDRICAL_SURFACE('',#29685,2.25);
#1609=CYLINDRICAL_SURFACE('',#29687,2.25);
#1610=CYLINDRICAL_SURFACE('',#29689,2.25);
#1611=CYLINDRICAL_SURFACE('',#29691,2.25);
#1612=CYLINDRICAL_SURFACE('',#29693,2.25);
#1613=CYLINDRICAL_SURFACE('',#29695,2.25);
#1614=CYLINDRICAL_SURFACE('',#29697,2.25);
#1615=CYLINDRICAL_SURFACE('',#29699,2.25);
#1616=CYLINDRICAL_SURFACE('',#29701,2.25);
#1617=CYLINDRICAL_SURFACE('',#29703,2.25);
#1618=CYLINDRICAL_SURFACE('',#29705,2.25);
#1619=CYLINDRICAL_SURFACE('',#29707,2.25);
#1620=CYLINDRICAL_SURFACE('',#29709,2.25);
#1621=CYLINDRICAL_SURFACE('',#29711,2.25);
#1622=CYLINDRICAL_SURFACE('',#29713,2.25);
#1623=CYLINDRICAL_SURFACE('',#29715,2.25);
#1624=CYLINDRICAL_SURFACE('',#29717,1.2866);
#1625=CYLINDRICAL_SURFACE('',#29719,1.486725);
#1626=CYLINDRICAL_SURFACE('',#29725,2.65);
#1627=CYLINDRICAL_SURFACE('',#29734,2.25);
#1928=FACE_BOUND('',#5395,.T.);
#1929=FACE_BOUND('',#5397,.T.);
#2316=CIRCLE('',#29537,1.486725);
#2317=CIRCLE('',#29542,1.486725);
#2318=CIRCLE('',#29544,1.2866);
#2319=CIRCLE('',#29551,2.25);
#2320=CIRCLE('',#29555,2.25);
#2321=CIRCLE('',#29559,2.25);
#2322=CIRCLE('',#29563,2.25);
#2323=CIRCLE('',#29567,2.25);
#2324=CIRCLE('',#29571,2.25);
#2325=CIRCLE('',#29572,2.25);
#2326=CIRCLE('',#29576,2.25);
#2327=CIRCLE('',#29580,2.25);
#2328=CIRCLE('',#29584,2.25);
#2329=CIRCLE('',#29588,2.25);
#2330=CIRCLE('',#29592,2.25);
#2331=CIRCLE('',#29596,2.25);
#2332=CIRCLE('',#29600,2.25);
#2333=CIRCLE('',#29604,2.25);
#2334=CIRCLE('',#29608,2.25);
#2335=CIRCLE('',#29612,2.25);
#2336=CIRCLE('',#29616,2.25);
#2337=CIRCLE('',#29620,2.25);
#2338=CIRCLE('',#29624,2.25);
#2339=CIRCLE('',#29628,2.25);
#2340=CIRCLE('',#29632,2.25);
#2341=CIRCLE('',#29636,2.25);
#2342=CIRCLE('',#29640,2.25);
#2343=CIRCLE('',#29644,2.25);
#2344=CIRCLE('',#29646,2.1);
#2345=CIRCLE('',#29647,2.25);
#2346=CIRCLE('',#29648,2.25);
#2347=CIRCLE('',#29649,2.25);
#2348=CIRCLE('',#29650,2.25);
#2349=CIRCLE('',#29651,2.25);
#2350=CIRCLE('',#29652,2.25);
#2351=CIRCLE('',#29653,2.25);
#2352=CIRCLE('',#29654,2.25);
#2353=CIRCLE('',#29655,2.25);
#2354=CIRCLE('',#29656,2.25);
#2355=CIRCLE('',#29657,2.25);
#2356=CIRCLE('',#29658,2.25);
#2357=CIRCLE('',#29659,2.25);
#2358=CIRCLE('',#29660,2.25);
#2359=CIRCLE('',#29661,2.25);
#2360=CIRCLE('',#29662,2.25);
#2361=CIRCLE('',#29663,2.25);
#2362=CIRCLE('',#29664,2.25);
#2363=CIRCLE('',#29665,2.25);
#2364=CIRCLE('',#29666,2.25);
#2365=CIRCLE('',#29667,2.25);
#2366=CIRCLE('',#29668,2.25);
#2367=CIRCLE('',#29669,2.25);
#2368=CIRCLE('',#29670,2.25);
#2369=CIRCLE('',#29672,2.25);
#2370=CIRCLE('',#29674,2.25);
#2371=CIRCLE('',#29676,2.25);
#2372=CIRCLE('',#29678,2.25);
#2373=CIRCLE('',#29680,2.25);
#2374=CIRCLE('',#29682,2.25);
#2375=CIRCLE('',#29684,2.25);
#2376=CIRCLE('',#29686,2.25);
#2377=CIRCLE('',#29688,2.25);
#2378=CIRCLE('',#29690,2.25);
#2379=CIRCLE('',#29692,2.25);
#2380=CIRCLE('',#29694,2.25);
#2381=CIRCLE('',#29696,2.25);
#2382=CIRCLE('',#29698,2.25);
#2383=CIRCLE('',#29700,2.25);
#2384=CIRCLE('',#29702,2.25);
#2385=CIRCLE('',#29704,2.25);
#2386=CIRCLE('',#29706,2.25);
#2387=CIRCLE('',#29708,2.25);
#2388=CIRCLE('',#29710,2.25);
#2389=CIRCLE('',#29712,2.25);
#2390=CIRCLE('',#29714,2.25);
#2391=CIRCLE('',#29716,2.25);
#2392=CIRCLE('',#29718,1.2866);
#2393=CIRCLE('',#29720,1.486725);
#2394=CIRCLE('',#29722,2.55);
#2395=CIRCLE('',#29724,2.65);
#2396=CIRCLE('',#29726,2.65);
#2397=CIRCLE('',#29728,2.5);
#2398=CIRCLE('',#29731,2.15);
#2399=CIRCLE('',#29733,2.25);
#2852=CONICAL_SURFACE('',#29645,2.175,0.785398163397429);
#2853=CONICAL_SURFACE('',#29723,2.6,0.785398163397477);
#2854=CONICAL_SURFACE('',#29727,2.575,0.785398163397429);
#2855=CONICAL_SURFACE('',#29732,2.2,0.785398163397477);
#3647=FACE_OUTER_BOUND('',#5281,.T.);
#3648=FACE_OUTER_BOUND('',#5282,.T.);
#3649=FACE_OUTER_BOUND('',#5283,.T.);
#3650=FACE_OUTER_BOUND('',#5284,.T.);
#3651=FACE_OUTER_BOUND('',#5285,.T.);
#3652=FACE_OUTER_BOUND('',#5286,.T.);
#3653=FACE_OUTER_BOUND('',#5287,.T.);
#3654=FACE_OUTER_BOUND('',#5288,.T.);
#3655=FACE_OUTER_BOUND('',#5289,.T.);
#3656=FACE_OUTER_BOUND('',#5290,.T.);
#3657=FACE_OUTER_BOUND('',#5291,.T.);
#3658=FACE_OUTER_BOUND('',#5292,.T.);
#3659=FACE_OUTER_BOUND('',#5293,.T.);
#3660=FACE_OUTER_BOUND('',#5294,.T.);
#3661=FACE_OUTER_BOUND('',#5295,.T.);
#3662=FACE_OUTER_BOUND('',#5296,.T.);
#3663=FACE_OUTER_BOUND('',#5297,.T.);
#3664=FACE_OUTER_BOUND('',#5298,.T.);
#3665=FACE_OUTER_BOUND('',#5299,.T.);
#3666=FACE_OUTER_BOUND('',#5300,.T.);
#3667=FACE_OUTER_BOUND('',#5301,.T.);
#3668=FACE_OUTER_BOUND('',#5302,.T.);
#3669=FACE_OUTER_BOUND('',#5303,.T.);
#3670=FACE_OUTER_BOUND('',#5304,.T.);
#3671=FACE_OUTER_BOUND('',#5305,.T.);
#3672=FACE_OUTER_BOUND('',#5306,.T.);
#3673=FACE_OUTER_BOUND('',#5307,.T.);
#3674=FACE_OUTER_BOUND('',#5308,.T.);
#3675=FACE_OUTER_BOUND('',#5309,.T.);
#3676=FACE_OUTER_BOUND('',#5310,.T.);
#3677=FACE_OUTER_BOUND('',#5311,.T.);
#3678=FACE_OUTER_BOUND('',#5312,.T.);
#3679=FACE_OUTER_BOUND('',#5313,.T.);
#3680=FACE_OUTER_BOUND('',#5314,.T.);
#3681=FACE_OUTER_BOUND('',#5315,.T.);
#3682=FACE_OUTER_BOUND('',#5316,.T.);
#3683=FACE_OUTER_BOUND('',#5317,.T.);
#3684=FACE_OUTER_BOUND('',#5318,.T.);
#3685=FACE_OUTER_BOUND('',#5319,.T.);
#3686=FACE_OUTER_BOUND('',#5320,.T.);
#3687=FACE_OUTER_BOUND('',#5321,.T.);
#3688=FACE_OUTER_BOUND('',#5322,.T.);
#3689=FACE_OUTER_BOUND('',#5323,.T.);
#3690=FACE_OUTER_BOUND('',#5324,.T.);
#3691=FACE_OUTER_BOUND('',#5325,.T.);
#3692=FACE_OUTER_BOUND('',#5326,.T.);
#3693=FACE_OUTER_BOUND('',#5327,.T.);
#3694=FACE_OUTER_BOUND('',#5328,.T.);
#3695=FACE_OUTER_BOUND('',#5329,.T.);
#3696=FACE_OUTER_BOUND('',#5330,.T.);
#3697=FACE_OUTER_BOUND('',#5331,.T.);
#3698=FACE_OUTER_BOUND('',#5332,.T.);
#3699=FACE_OUTER_BOUND('',#5333,.T.);
#3700=FACE_OUTER_BOUND('',#5334,.T.);
#3701=FACE_OUTER_BOUND('',#5335,.T.);
#3702=FACE_OUTER_BOUND('',#5336,.T.);
#3703=FACE_OUTER_BOUND('',#5337,.T.);
#3704=FACE_OUTER_BOUND('',#5338,.T.);
#3705=FACE_OUTER_BOUND('',#5339,.T.);
#3706=FACE_OUTER_BOUND('',#5340,.T.);
#3707=FACE_OUTER_BOUND('',#5341,.T.);
#3708=FACE_OUTER_BOUND('',#5342,.T.);
#3709=FACE_OUTER_BOUND('',#5343,.T.);
#3710=FACE_OUTER_BOUND('',#5344,.T.);
#3711=FACE_OUTER_BOUND('',#5345,.T.);
#3712=FACE_OUTER_BOUND('',#5346,.T.);
#3713=FACE_OUTER_BOUND('',#5347,.T.);
#3714=FACE_OUTER_BOUND('',#5348,.T.);
#3715=FACE_OUTER_BOUND('',#5349,.T.);
#3716=FACE_OUTER_BOUND('',#5350,.T.);
#3717=FACE_OUTER_BOUND('',#5351,.T.);
#3718=FACE_OUTER_BOUND('',#5352,.T.);
#3719=FACE_OUTER_BOUND('',#5353,.T.);
#3720=FACE_OUTER_BOUND('',#5354,.T.);
#3721=FACE_OUTER_BOUND('',#5355,.T.);
#3722=FACE_OUTER_BOUND('',#5356,.T.);
#3723=FACE_OUTER_BOUND('',#5357,.T.);
#3724=FACE_OUTER_BOUND('',#5358,.T.);
#3725=FACE_OUTER_BOUND('',#5359,.T.);
#3726=FACE_OUTER_BOUND('',#5360,.T.);
#3727=FACE_OUTER_BOUND('',#5361,.T.);
#3728=FACE_OUTER_BOUND('',#5362,.T.);
#3729=FACE_OUTER_BOUND('',#5363,.T.);
#3730=FACE_OUTER_BOUND('',#5364,.T.);
#3731=FACE_OUTER_BOUND('',#5365,.T.);
#3732=FACE_OUTER_BOUND('',#5366,.T.);
#3733=FACE_OUTER_BOUND('',#5367,.T.);
#3734=FACE_OUTER_BOUND('',#5368,.T.);
#3735=FACE_OUTER_BOUND('',#5369,.T.);
#3736=FACE_OUTER_BOUND('',#5370,.T.);
#3737=FACE_OUTER_BOUND('',#5371,.T.);
#3738=FACE_OUTER_BOUND('',#5372,.T.);
#3739=FACE_OUTER_BOUND('',#5373,.T.);
#3740=FACE_OUTER_BOUND('',#5374,.T.);
#3741=FACE_OUTER_BOUND('',#5375,.T.);
#3742=FACE_OUTER_BOUND('',#5376,.T.);
#3743=FACE_OUTER_BOUND('',#5377,.T.);
#3744=FACE_OUTER_BOUND('',#5378,.T.);
#3745=FACE_OUTER_BOUND('',#5379,.T.);
#3746=FACE_OUTER_BOUND('',#5380,.T.);
#3747=FACE_OUTER_BOUND('',#5381,.T.);
#3748=FACE_OUTER_BOUND('',#5382,.T.);
#3749=FACE_OUTER_BOUND('',#5383,.T.);
#3750=FACE_OUTER_BOUND('',#5384,.T.);
#3751=FACE_OUTER_BOUND('',#5385,.T.);
#3752=FACE_OUTER_BOUND('',#5386,.T.);
#3753=FACE_OUTER_BOUND('',#5387,.T.);
#3754=FACE_OUTER_BOUND('',#5388,.T.);
#3755=FACE_OUTER_BOUND('',#5389,.T.);
#3756=FACE_OUTER_BOUND('',#5390,.T.);
#3757=FACE_OUTER_BOUND('',#5391,.T.);
#3758=FACE_OUTER_BOUND('',#5392,.T.);
#3759=FACE_OUTER_BOUND('',#5393,.T.);
#3760=FACE_OUTER_BOUND('',#5394,.T.);
#3761=FACE_OUTER_BOUND('',#5396,.T.);
#3762=FACE_OUTER_BOUND('',#5398,.T.);
#3763=FACE_OUTER_BOUND('',#5399,.T.);
#3764=FACE_OUTER_BOUND('',#5400,.T.);
#5281=EDGE_LOOP('',(#21451,#21452,#21453,#21454));
#5282=EDGE_LOOP('',(#21455,#21456,#21457,#21458));
#5283=EDGE_LOOP('',(#21459,#21460,#21461,#21462));
#5284=EDGE_LOOP('',(#21463,#21464,#21465,#21466));
#5285=EDGE_LOOP('',(#21467,#21468,#21469,#21470,#21471));
#5286=EDGE_LOOP('',(#21472,#21473,#21474,#21475));
#5287=EDGE_LOOP('',(#21476,#21477,#21478,#21479));
#5288=EDGE_LOOP('',(#21480,#21481,#21482,#21483));
#5289=EDGE_LOOP('',(#21484,#21485,#21486,#21487));
#5290=EDGE_LOOP('',(#21488,#21489,#21490,#21491));
#5291=EDGE_LOOP('',(#21492,#21493,#21494,#21495));
#5292=EDGE_LOOP('',(#21496,#21497,#21498));
#5293=EDGE_LOOP('',(#21499,#21500,#21501,#21502));
#5294=EDGE_LOOP('',(#21503,#21504,#21505,#21506));
#5295=EDGE_LOOP('',(#21507,#21508,#21509));
#5296=EDGE_LOOP('',(#21510,#21511,#21512,#21513));
#5297=EDGE_LOOP('',(#21514,#21515,#21516,#21517));
#5298=EDGE_LOOP('',(#21518,#21519,#21520));
#5299=EDGE_LOOP('',(#21521,#21522,#21523,#21524));
#5300=EDGE_LOOP('',(#21525,#21526,#21527,#21528));
#5301=EDGE_LOOP('',(#21529,#21530,#21531));
#5302=EDGE_LOOP('',(#21532,#21533,#21534,#21535));
#5303=EDGE_LOOP('',(#21536,#21537,#21538,#21539));
#5304=EDGE_LOOP('',(#21540,#21541,#21542));
#5305=EDGE_LOOP('',(#21543,#21544,#21545,#21546));
#5306=EDGE_LOOP('',(#21547,#21548,#21549,#21550));
#5307=EDGE_LOOP('',(#21551,#21552,#21553,#21554));
#5308=EDGE_LOOP('',(#21555,#21556,#21557,#21558));
#5309=EDGE_LOOP('',(#21559,#21560,#21561,#21562));
#5310=EDGE_LOOP('',(#21563,#21564,#21565));
#5311=EDGE_LOOP('',(#21566,#21567,#21568,#21569));
#5312=EDGE_LOOP('',(#21570,#21571,#21572,#21573));
#5313=EDGE_LOOP('',(#21574,#21575,#21576));
#5314=EDGE_LOOP('',(#21577,#21578,#21579,#21580));
#5315=EDGE_LOOP('',(#21581,#21582,#21583,#21584));
#5316=EDGE_LOOP('',(#21585,#21586,#21587));
#5317=EDGE_LOOP('',(#21588,#21589,#21590,#21591));
#5318=EDGE_LOOP('',(#21592,#21593,#21594,#21595));
#5319=EDGE_LOOP('',(#21596,#21597,#21598));
#5320=EDGE_LOOP('',(#21599,#21600,#21601,#21602));
#5321=EDGE_LOOP('',(#21603,#21604,#21605,#21606));
#5322=EDGE_LOOP('',(#21607,#21608,#21609));
#5323=EDGE_LOOP('',(#21610,#21611,#21612,#21613));
#5324=EDGE_LOOP('',(#21614,#21615,#21616,#21617));
#5325=EDGE_LOOP('',(#21618,#21619,#21620));
#5326=EDGE_LOOP('',(#21621,#21622,#21623,#21624));
#5327=EDGE_LOOP('',(#21625,#21626,#21627,#21628));
#5328=EDGE_LOOP('',(#21629,#21630,#21631));
#5329=EDGE_LOOP('',(#21632,#21633,#21634,#21635));
#5330=EDGE_LOOP('',(#21636,#21637,#21638,#21639));
#5331=EDGE_LOOP('',(#21640,#21641,#21642));
#5332=EDGE_LOOP('',(#21643,#21644,#21645,#21646));
#5333=EDGE_LOOP('',(#21647,#21648,#21649,#21650));
#5334=EDGE_LOOP('',(#21651,#21652,#21653));
#5335=EDGE_LOOP('',(#21654,#21655,#21656,#21657));
#5336=EDGE_LOOP('',(#21658,#21659,#21660,#21661));
#5337=EDGE_LOOP('',(#21662,#21663,#21664));
#5338=EDGE_LOOP('',(#21665,#21666,#21667,#21668));
#5339=EDGE_LOOP('',(#21669,#21670,#21671,#21672));
#5340=EDGE_LOOP('',(#21673,#21674,#21675));
#5341=EDGE_LOOP('',(#21676,#21677,#21678,#21679));
#5342=EDGE_LOOP('',(#21680,#21681,#21682,#21683));
#5343=EDGE_LOOP('',(#21684,#21685,#21686));
#5344=EDGE_LOOP('',(#21687,#21688,#21689,#21690));
#5345=EDGE_LOOP('',(#21691,#21692,#21693,#21694));
#5346=EDGE_LOOP('',(#21695,#21696,#21697));
#5347=EDGE_LOOP('',(#21698,#21699,#21700,#21701));
#5348=EDGE_LOOP('',(#21702,#21703,#21704,#21705));
#5349=EDGE_LOOP('',(#21706,#21707,#21708));
#5350=EDGE_LOOP('',(#21709,#21710,#21711,#21712));
#5351=EDGE_LOOP('',(#21713,#21714,#21715,#21716));
#5352=EDGE_LOOP('',(#21717,#21718,#21719));
#5353=EDGE_LOOP('',(#21720,#21721,#21722,#21723));
#5354=EDGE_LOOP('',(#21724,#21725,#21726,#21727));
#5355=EDGE_LOOP('',(#21728,#21729,#21730));
#5356=EDGE_LOOP('',(#21731,#21732,#21733,#21734));
#5357=EDGE_LOOP('',(#21735,#21736,#21737,#21738));
#5358=EDGE_LOOP('',(#21739,#21740,#21741));
#5359=EDGE_LOOP('',(#21742,#21743,#21744,#21745));
#5360=EDGE_LOOP('',(#21746,#21747,#21748,#21749));
#5361=EDGE_LOOP('',(#21750,#21751,#21752));
#5362=EDGE_LOOP('',(#21753,#21754,#21755,#21756,#21757,#21758,#21759,#21760,
#21761,#21762,#21763,#21764,#21765,#21766,#21767,#21768,#21769,#21770,#21771,
#21772,#21773,#21774,#21775,#21776,#21777,#21778,#21779,#21780,#21781,#21782,
#21783,#21784,#21785,#21786,#21787,#21788,#21789,#21790,#21791,#21792,#21793,
#21794,#21795,#21796,#21797,#21798,#21799,#21800,#21801,#21802,#21803,#21804,
#21805,#21806,#21807,#21808,#21809,#21810,#21811,#21812,#21813,#21814,#21815,
#21816,#21817,#21818,#21819,#21820,#21821,#21822,#21823,#21824,#21825,#21826,
#21827));
#5363=EDGE_LOOP('',(#21828,#21829,#21830,#21831));
#5364=EDGE_LOOP('',(#21832,#21833,#21834,#21835));
#5365=EDGE_LOOP('',(#21836,#21837,#21838,#21839));
#5366=EDGE_LOOP('',(#21840,#21841,#21842,#21843));
#5367=EDGE_LOOP('',(#21844,#21845,#21846,#21847));
#5368=EDGE_LOOP('',(#21848,#21849,#21850,#21851));
#5369=EDGE_LOOP('',(#21852,#21853,#21854,#21855));
#5370=EDGE_LOOP('',(#21856,#21857,#21858,#21859));
#5371=EDGE_LOOP('',(#21860,#21861,#21862,#21863));
#5372=EDGE_LOOP('',(#21864,#21865,#21866,#21867));
#5373=EDGE_LOOP('',(#21868,#21869,#21870,#21871));
#5374=EDGE_LOOP('',(#21872,#21873,#21874,#21875));
#5375=EDGE_LOOP('',(#21876,#21877,#21878,#21879));
#5376=EDGE_LOOP('',(#21880,#21881,#21882,#21883));
#5377=EDGE_LOOP('',(#21884,#21885,#21886,#21887));
#5378=EDGE_LOOP('',(#21888,#21889,#21890,#21891));
#5379=EDGE_LOOP('',(#21892,#21893,#21894,#21895));
#5380=EDGE_LOOP('',(#21896,#21897,#21898,#21899));
#5381=EDGE_LOOP('',(#21900,#21901,#21902,#21903));
#5382=EDGE_LOOP('',(#21904,#21905,#21906,#21907));
#5383=EDGE_LOOP('',(#21908,#21909,#21910,#21911));
#5384=EDGE_LOOP('',(#21912,#21913,#21914,#21915));
#5385=EDGE_LOOP('',(#21916,#21917,#21918,#21919));
#5386=EDGE_LOOP('',(#21920,#21921,#21922,#21923,#21924,#21925,#21926,#21927,
#21928,#21929,#21930,#21931,#21932));
#5387=EDGE_LOOP('',(#21933,#21934,#21935,#21936));
#5388=EDGE_LOOP('',(#21937,#21938,#21939,#21940,#21941,#21942,#21943,#21944,
#21945,#21946,#21947,#21948));
#5389=EDGE_LOOP('',(#21949,#21950,#21951));
#5390=EDGE_LOOP('',(#21952));
#5391=EDGE_LOOP('',(#21953,#21954,#21955,#21956));
#5392=EDGE_LOOP('',(#21957,#21958,#21959,#21960));
#5393=EDGE_LOOP('',(#21961,#21962,#21963,#21964));
#5394=EDGE_LOOP('',(#21965));
#5395=EDGE_LOOP('',(#21966,#21967,#21968,#21969));
#5396=EDGE_LOOP('',(#21970));
#5397=EDGE_LOOP('',(#21971,#21972,#21973,#21974,#21975));
#5398=EDGE_LOOP('',(#21976,#21977,#21978,#21979,#21980,#21981,#21982,#21983,
#21984,#21985,#21986,#21987,#21988,#21989,#21990,#21991,#21992,#21993,#21994,
#21995,#21996,#21997,#21998,#21999,#22000,#22001,#22002,#22003,#22004,#22005,
#22006,#22007,#22008,#22009,#22010,#22011,#22012,#22013,#22014,#22015,#22016,
#22017,#22018,#22019,#22020,#22021,#22022,#22023,#22024,#22025,#22026,#22027));
#5399=EDGE_LOOP('',(#22028,#22029,#22030,#22031));
#5400=EDGE_LOOP('',(#22032));
#7563=LINE('',#44022,#10051);
#7564=LINE('',#44055,#10052);
#7565=LINE('',#44145,#10053);
#7566=LINE('',#44235,#10054);
#7567=LINE('',#44325,#10055);
#7568=LINE('',#44414,#10056);
#7569=LINE('',#44442,#10057);
#7570=LINE('',#44480,#10058);
#7571=LINE('',#44518,#10059);
#7572=LINE('',#44556,#10060);
#7573=LINE('',#44558,#10061);
#7574=LINE('',#44560,#10062);
#7575=LINE('',#44570,#10063);
#7576=LINE('',#44571,#10064);
#7577=LINE('',#44577,#10065);
#7578=LINE('',#44579,#10066);
#7579=LINE('',#44581,#10067);
#7580=LINE('',#44591,#10068);
#7581=LINE('',#44592,#10069);
#7582=LINE('',#44598,#10070);
#7583=LINE('',#44600,#10071);
#7584=LINE('',#44602,#10072);
#7585=LINE('',#44612,#10073);
#7586=LINE('',#44613,#10074);
#7587=LINE('',#44619,#10075);
#7588=LINE('',#44621,#10076);
#7589=LINE('',#44623,#10077);
#7590=LINE('',#44633,#10078);
#7591=LINE('',#44634,#10079);
#7592=LINE('',#44640,#10080);
#7593=LINE('',#44642,#10081);
#7594=LINE('',#44644,#10082);
#7595=LINE('',#44654,#10083);
#7596=LINE('',#44655,#10084);
#7597=LINE('',#44661,#10085);
#7598=LINE('',#44663,#10086);
#7599=LINE('',#44665,#10087);
#7600=LINE('',#44675,#10088);
#7601=LINE('',#44676,#10089);
#7602=LINE('',#44684,#10090);
#7603=LINE('',#44686,#10091);
#7604=LINE('',#44688,#10092);
#7605=LINE('',#44698,#10093);
#7606=LINE('',#44699,#10094);
#7607=LINE('',#44705,#10095);
#7608=LINE('',#44707,#10096);
#7609=LINE('',#44709,#10097);
#7610=LINE('',#44719,#10098);
#7611=LINE('',#44720,#10099);
#7612=LINE('',#44726,#10100);
#7613=LINE('',#44728,#10101);
#7614=LINE('',#44730,#10102);
#7615=LINE('',#44740,#10103);
#7616=LINE('',#44741,#10104);
#7617=LINE('',#44747,#10105);
#7618=LINE('',#44749,#10106);
#7619=LINE('',#44751,#10107);
#7620=LINE('',#44761,#10108);
#7621=LINE('',#44762,#10109);
#7622=LINE('',#44768,#10110);
#7623=LINE('',#44770,#10111);
#7624=LINE('',#44772,#10112);
#7625=LINE('',#44782,#10113);
#7626=LINE('',#44783,#10114);
#7627=LINE('',#44789,#10115);
#7628=LINE('',#44791,#10116);
#7629=LINE('',#44793,#10117);
#7630=LINE('',#44803,#10118);
#7631=LINE('',#44804,#10119);
#7632=LINE('',#44810,#10120);
#7633=LINE('',#44812,#10121);
#7634=LINE('',#44814,#10122);
#7635=LINE('',#44824,#10123);
#7636=LINE('',#44825,#10124);
#7637=LINE('',#44831,#10125);
#7638=LINE('',#44833,#10126);
#7639=LINE('',#44835,#10127);
#7640=LINE('',#44845,#10128);
#7641=LINE('',#44846,#10129);
#7642=LINE('',#44852,#10130);
#7643=LINE('',#44854,#10131);
#7644=LINE('',#44856,#10132);
#7645=LINE('',#44866,#10133);
#7646=LINE('',#44867,#10134);
#7647=LINE('',#44873,#10135);
#7648=LINE('',#44875,#10136);
#7649=LINE('',#44877,#10137);
#7650=LINE('',#44887,#10138);
#7651=LINE('',#44888,#10139);
#7652=LINE('',#44894,#10140);
#7653=LINE('',#44896,#10141);
#7654=LINE('',#44898,#10142);
#7655=LINE('',#44908,#10143);
#7656=LINE('',#44909,#10144);
#7657=LINE('',#44915,#10145);
#7658=LINE('',#44917,#10146);
#7659=LINE('',#44919,#10147);
#7660=LINE('',#44929,#10148);
#7661=LINE('',#44930,#10149);
#7662=LINE('',#44936,#10150);
#7663=LINE('',#44938,#10151);
#7664=LINE('',#44940,#10152);
#7665=LINE('',#44950,#10153);
#7666=LINE('',#44951,#10154);
#7667=LINE('',#44957,#10155);
#7668=LINE('',#44959,#10156);
#7669=LINE('',#44961,#10157);
#7670=LINE('',#44971,#10158);
#7671=LINE('',#44972,#10159);
#7672=LINE('',#44978,#10160);
#7673=LINE('',#44980,#10161);
#7674=LINE('',#44982,#10162);
#7675=LINE('',#44992,#10163);
#7676=LINE('',#44993,#10164);
#7677=LINE('',#44999,#10165);
#7678=LINE('',#45001,#10166);
#7679=LINE('',#45003,#10167);
#7680=LINE('',#45013,#10168);
#7681=LINE('',#45014,#10169);
#7682=LINE('',#45020,#10170);
#7683=LINE('',#45022,#10171);
#7684=LINE('',#45024,#10172);
#7685=LINE('',#45034,#10173);
#7686=LINE('',#45035,#10174);
#7687=LINE('',#45041,#10175);
#7688=LINE('',#45043,#10176);
#7689=LINE('',#45045,#10177);
#7690=LINE('',#45055,#10178);
#7691=LINE('',#45056,#10179);
#7692=LINE('',#45062,#10180);
#7693=LINE('',#46048,#10181);
#7694=LINE('',#46052,#10182);
#7695=LINE('',#46056,#10183);
#7696=LINE('',#46063,#10184);
#10051=VECTOR('',#33814,1.5);
#10052=VECTOR('',#33819,1.5);
#10053=VECTOR('',#33822,1.5);
#10054=VECTOR('',#33825,1.5);
#10055=VECTOR('',#33828,1.5);
#10056=VECTOR('',#33833,1.2866);
#10057=VECTOR('',#33838,1.2866);
#10058=VECTOR('',#33841,1.2866);
#10059=VECTOR('',#33844,1.2866);
#10060=VECTOR('',#33847,1.);
#10061=VECTOR('',#33848,1.);
#10062=VECTOR('',#33849,1.);
#10063=VECTOR('',#33852,1.);
#10064=VECTOR('',#33853,1.);
#10065=VECTOR('',#33860,1.);
#10066=VECTOR('',#33861,1.);
#10067=VECTOR('',#33862,1.);
#10068=VECTOR('',#33865,1.);
#10069=VECTOR('',#33866,1.);
#10070=VECTOR('',#33873,1.);
#10071=VECTOR('',#33874,1.);
#10072=VECTOR('',#33875,1.);
#10073=VECTOR('',#33878,1.);
#10074=VECTOR('',#33879,1.);
#10075=VECTOR('',#33886,1.);
#10076=VECTOR('',#33887,1.);
#10077=VECTOR('',#33888,1.);
#10078=VECTOR('',#33891,1.);
#10079=VECTOR('',#33892,1.);
#10080=VECTOR('',#33899,1.);
#10081=VECTOR('',#33900,1.);
#10082=VECTOR('',#33901,1.);
#10083=VECTOR('',#33904,1.);
#10084=VECTOR('',#33905,1.);
#10085=VECTOR('',#33912,1.);
#10086=VECTOR('',#33913,1.);
#10087=VECTOR('',#33914,1.);
#10088=VECTOR('',#33917,1.);
#10089=VECTOR('',#33918,1.);
#10090=VECTOR('',#33927,1.);
#10091=VECTOR('',#33928,1.);
#10092=VECTOR('',#33929,1.);
#10093=VECTOR('',#33932,1.);
#10094=VECTOR('',#33933,1.);
#10095=VECTOR('',#33940,1.);
#10096=VECTOR('',#33941,1.);
#10097=VECTOR('',#33942,1.);
#10098=VECTOR('',#33945,1.);
#10099=VECTOR('',#33946,1.);
#10100=VECTOR('',#33953,1.);
#10101=VECTOR('',#33954,1.);
#10102=VECTOR('',#33955,1.);
#10103=VECTOR('',#33958,1.);
#10104=VECTOR('',#33959,1.);
#10105=VECTOR('',#33966,1.);
#10106=VECTOR('',#33967,1.);
#10107=VECTOR('',#33968,1.);
#10108=VECTOR('',#33971,1.);
#10109=VECTOR('',#33972,1.);
#10110=VECTOR('',#33979,1.);
#10111=VECTOR('',#33980,1.);
#10112=VECTOR('',#33981,1.);
#10113=VECTOR('',#33984,1.);
#10114=VECTOR('',#33985,1.);
#10115=VECTOR('',#33992,1.);
#10116=VECTOR('',#33993,1.);
#10117=VECTOR('',#33994,1.);
#10118=VECTOR('',#33997,1.);
#10119=VECTOR('',#33998,1.);
#10120=VECTOR('',#34005,1.);
#10121=VECTOR('',#34006,1.);
#10122=VECTOR('',#34007,1.);
#10123=VECTOR('',#34010,1.);
#10124=VECTOR('',#34011,1.);
#10125=VECTOR('',#34018,1.);
#10126=VECTOR('',#34019,1.);
#10127=VECTOR('',#34020,1.);
#10128=VECTOR('',#34023,1.);
#10129=VECTOR('',#34024,1.);
#10130=VECTOR('',#34031,1.);
#10131=VECTOR('',#34032,1.);
#10132=VECTOR('',#34033,1.);
#10133=VECTOR('',#34036,1.);
#10134=VECTOR('',#34037,1.);
#10135=VECTOR('',#34044,1.);
#10136=VECTOR('',#34045,1.);
#10137=VECTOR('',#34046,1.);
#10138=VECTOR('',#34049,1.);
#10139=VECTOR('',#34050,1.);
#10140=VECTOR('',#34057,1.);
#10141=VECTOR('',#34058,1.);
#10142=VECTOR('',#34059,1.);
#10143=VECTOR('',#34062,1.);
#10144=VECTOR('',#34063,1.);
#10145=VECTOR('',#34070,1.);
#10146=VECTOR('',#34071,1.);
#10147=VECTOR('',#34072,1.);
#10148=VECTOR('',#34075,1.);
#10149=VECTOR('',#34076,1.);
#10150=VECTOR('',#34083,1.);
#10151=VECTOR('',#34084,1.);
#10152=VECTOR('',#34085,1.);
#10153=VECTOR('',#34088,1.);
#10154=VECTOR('',#34089,1.);
#10155=VECTOR('',#34096,1.);
#10156=VECTOR('',#34097,1.);
#10157=VECTOR('',#34098,1.);
#10158=VECTOR('',#34101,1.);
#10159=VECTOR('',#34102,1.);
#10160=VECTOR('',#34109,1.);
#10161=VECTOR('',#34110,1.);
#10162=VECTOR('',#34111,1.);
#10163=VECTOR('',#34114,1.);
#10164=VECTOR('',#34115,1.);
#10165=VECTOR('',#34122,1.);
#10166=VECTOR('',#34123,1.);
#10167=VECTOR('',#34124,1.);
#10168=VECTOR('',#34127,1.);
#10169=VECTOR('',#34128,1.);
#10170=VECTOR('',#34135,1.);
#10171=VECTOR('',#34136,1.);
#10172=VECTOR('',#34137,1.);
#10173=VECTOR('',#34140,1.);
#10174=VECTOR('',#34141,1.);
#10175=VECTOR('',#34148,1.);
#10176=VECTOR('',#34149,1.);
#10177=VECTOR('',#34150,1.);
#10178=VECTOR('',#34153,1.);
#10179=VECTOR('',#34154,1.);
#10180=VECTOR('',#34163,2.175);
#10181=VECTOR('',#34320,2.6);
#10182=VECTOR('',#34325,2.65);
#10183=VECTOR('',#34330,2.575);
#10184=VECTOR('',#34341,2.2);
#12374=VERTEX_POINT('',#44020);
#12375=VERTEX_POINT('',#44021);
#12376=VERTEX_POINT('',#44023);
#12377=VERTEX_POINT('',#44040);
#12378=VERTEX_POINT('',#44053);
#12379=VERTEX_POINT('',#44054);
#12380=VERTEX_POINT('',#44143);
#12381=VERTEX_POINT('',#44144);
#12382=VERTEX_POINT('',#44233);
#12383=VERTEX_POINT('',#44234);
#12384=VERTEX_POINT('',#44323);
#12385=VERTEX_POINT('',#44324);
#12386=VERTEX_POINT('',#44326);
#12387=VERTEX_POINT('',#44412);
#12388=VERTEX_POINT('',#44413);
#12389=VERTEX_POINT('',#44415);
#12390=VERTEX_POINT('',#44428);
#12391=VERTEX_POINT('',#44440);
#12392=VERTEX_POINT('',#44441);
#12393=VERTEX_POINT('',#44478);
#12394=VERTEX_POINT('',#44479);
#12395=VERTEX_POINT('',#44516);
#12396=VERTEX_POINT('',#44517);
#12397=VERTEX_POINT('',#44554);
#12398=VERTEX_POINT('',#44555);
#12399=VERTEX_POINT('',#44557);
#12400=VERTEX_POINT('',#44559);
#12401=VERTEX_POINT('',#44565);
#12402=VERTEX_POINT('',#44569);
#12403=VERTEX_POINT('',#44575);
#12404=VERTEX_POINT('',#44576);
#12405=VERTEX_POINT('',#44578);
#12406=VERTEX_POINT('',#44580);
#12407=VERTEX_POINT('',#44586);
#12408=VERTEX_POINT('',#44590);
#12409=VERTEX_POINT('',#44596);
#12410=VERTEX_POINT('',#44597);
#12411=VERTEX_POINT('',#44599);
#12412=VERTEX_POINT('',#44601);
#12413=VERTEX_POINT('',#44607);
#12414=VERTEX_POINT('',#44611);
#12415=VERTEX_POINT('',#44617);
#12416=VERTEX_POINT('',#44618);
#12417=VERTEX_POINT('',#44620);
#12418=VERTEX_POINT('',#44622);
#12419=VERTEX_POINT('',#44628);
#12420=VERTEX_POINT('',#44632);
#12421=VERTEX_POINT('',#44638);
#12422=VERTEX_POINT('',#44639);
#12423=VERTEX_POINT('',#44641);
#12424=VERTEX_POINT('',#44643);
#12425=VERTEX_POINT('',#44649);
#12426=VERTEX_POINT('',#44653);
#12427=VERTEX_POINT('',#44659);
#12428=VERTEX_POINT('',#44660);
#12429=VERTEX_POINT('',#44662);
#12430=VERTEX_POINT('',#44664);
#12431=VERTEX_POINT('',#44670);
#12432=VERTEX_POINT('',#44674);
#12433=VERTEX_POINT('',#44678);
#12434=VERTEX_POINT('',#44682);
#12435=VERTEX_POINT('',#44683);
#12436=VERTEX_POINT('',#44685);
#12437=VERTEX_POINT('',#44687);
#12438=VERTEX_POINT('',#44693);
#12439=VERTEX_POINT('',#44697);
#12440=VERTEX_POINT('',#44703);
#12441=VERTEX_POINT('',#44704);
#12442=VERTEX_POINT('',#44706);
#12443=VERTEX_POINT('',#44708);
#12444=VERTEX_POINT('',#44714);
#12445=VERTEX_POINT('',#44718);
#12446=VERTEX_POINT('',#44724);
#12447=VERTEX_POINT('',#44725);
#12448=VERTEX_POINT('',#44727);
#12449=VERTEX_POINT('',#44729);
#12450=VERTEX_POINT('',#44735);
#12451=VERTEX_POINT('',#44739);
#12452=VERTEX_POINT('',#44745);
#12453=VERTEX_POINT('',#44746);
#12454=VERTEX_POINT('',#44748);
#12455=VERTEX_POINT('',#44750);
#12456=VERTEX_POINT('',#44756);
#12457=VERTEX_POINT('',#44760);
#12458=VERTEX_POINT('',#44766);
#12459=VERTEX_POINT('',#44767);
#12460=VERTEX_POINT('',#44769);
#12461=VERTEX_POINT('',#44771);
#12462=VERTEX_POINT('',#44777);
#12463=VERTEX_POINT('',#44781);
#12464=VERTEX_POINT('',#44787);
#12465=VERTEX_POINT('',#44788);
#12466=VERTEX_POINT('',#44790);
#12467=VERTEX_POINT('',#44792);
#12468=VERTEX_POINT('',#44798);
#12469=VERTEX_POINT('',#44802);
#12470=VERTEX_POINT('',#44808);
#12471=VERTEX_POINT('',#44809);
#12472=VERTEX_POINT('',#44811);
#12473=VERTEX_POINT('',#44813);
#12474=VERTEX_POINT('',#44819);
#12475=VERTEX_POINT('',#44823);
#12476=VERTEX_POINT('',#44829);
#12477=VERTEX_POINT('',#44830);
#12478=VERTEX_POINT('',#44832);
#12479=VERTEX_POINT('',#44834);
#12480=VERTEX_POINT('',#44840);
#12481=VERTEX_POINT('',#44844);
#12482=VERTEX_POINT('',#44850);
#12483=VERTEX_POINT('',#44851);
#12484=VERTEX_POINT('',#44853);
#12485=VERTEX_POINT('',#44855);
#12486=VERTEX_POINT('',#44861);
#12487=VERTEX_POINT('',#44865);
#12488=VERTEX_POINT('',#44871);
#12489=VERTEX_POINT('',#44872);
#12490=VERTEX_POINT('',#44874);
#12491=VERTEX_POINT('',#44876);
#12492=VERTEX_POINT('',#44882);
#12493=VERTEX_POINT('',#44886);
#12494=VERTEX_POINT('',#44892);
#12495=VERTEX_POINT('',#44893);
#12496=VERTEX_POINT('',#44895);
#12497=VERTEX_POINT('',#44897);
#12498=VERTEX_POINT('',#44903);
#12499=VERTEX_POINT('',#44907);
#12500=VERTEX_POINT('',#44913);
#12501=VERTEX_POINT('',#44914);
#12502=VERTEX_POINT('',#44916);
#12503=VERTEX_POINT('',#44918);
#12504=VERTEX_POINT('',#44924);
#12505=VERTEX_POINT('',#44928);
#12506=VERTEX_POINT('',#44934);
#12507=VERTEX_POINT('',#44935);
#12508=VERTEX_POINT('',#44937);
#12509=VERTEX_POINT('',#44939);
#12510=VERTEX_POINT('',#44945);
#12511=VERTEX_POINT('',#44949);
#12512=VERTEX_POINT('',#44955);
#12513=VERTEX_POINT('',#44956);
#12514=VERTEX_POINT('',#44958);
#12515=VERTEX_POINT('',#44960);
#12516=VERTEX_POINT('',#44966);
#12517=VERTEX_POINT('',#44970);
#12518=VERTEX_POINT('',#44976);
#12519=VERTEX_POINT('',#44977);
#12520=VERTEX_POINT('',#44979);
#12521=VERTEX_POINT('',#44981);
#12522=VERTEX_POINT('',#44987);
#12523=VERTEX_POINT('',#44991);
#12524=VERTEX_POINT('',#44997);
#12525=VERTEX_POINT('',#44998);
#12526=VERTEX_POINT('',#45000);
#12527=VERTEX_POINT('',#45002);
#12528=VERTEX_POINT('',#45008);
#12529=VERTEX_POINT('',#45012);
#12530=VERTEX_POINT('',#45018);
#12531=VERTEX_POINT('',#45019);
#12532=VERTEX_POINT('',#45021);
#12533=VERTEX_POINT('',#45023);
#12534=VERTEX_POINT('',#45029);
#12535=VERTEX_POINT('',#45033);
#12536=VERTEX_POINT('',#45039);
#12537=VERTEX_POINT('',#45040);
#12538=VERTEX_POINT('',#45042);
#12539=VERTEX_POINT('',#45044);
#12540=VERTEX_POINT('',#45050);
#12541=VERTEX_POINT('',#45054);
#12542=VERTEX_POINT('',#45060);
#12543=VERTEX_POINT('',#45385);
#12544=VERTEX_POINT('',#45484);
#12545=VERTEX_POINT('',#45592);
#12546=VERTEX_POINT('',#46043);
#12547=VERTEX_POINT('',#46046);
#12548=VERTEX_POINT('',#46050);
#12549=VERTEX_POINT('',#46054);
#12550=VERTEX_POINT('',#46059);
#15609=EDGE_CURVE('',#12374,#12375,#7563,.T.);
#15610=EDGE_CURVE('',#12374,#12376,#785,.T.);
#15611=EDGE_CURVE('',#12376,#12377,#2316,.F.);
#15612=EDGE_CURVE('',#12377,#12375,#786,.T.);
#15613=EDGE_CURVE('',#12378,#12379,#7564,.T.);
#15614=EDGE_CURVE('',#12378,#12374,#787,.T.);
#15615=EDGE_CURVE('',#12375,#12379,#788,.T.);
#15616=EDGE_CURVE('',#12380,#12381,#7565,.T.);
#15617=EDGE_CURVE('',#12380,#12378,#789,.T.);
#15618=EDGE_CURVE('',#12379,#12381,#790,.T.);
#15619=EDGE_CURVE('',#12382,#12383,#7566,.T.);
#15620=EDGE_CURVE('',#12382,#12380,#791,.T.);
#15621=EDGE_CURVE('',#12381,#12383,#792,.T.);
#15622=EDGE_CURVE('',#12384,#12385,#7567,.T.);
#15623=EDGE_CURVE('',#12386,#12384,#2317,.T.);
#15624=EDGE_CURVE('',#12386,#12382,#793,.T.);
#15625=EDGE_CURVE('',#12383,#12385,#794,.T.);
#15626=EDGE_CURVE('',#12387,#12388,#7568,.T.);
#15627=EDGE_CURVE('',#12387,#12389,#795,.T.);
#15628=EDGE_CURVE('',#12390,#12389,#2318,.T.);
#15629=EDGE_CURVE('',#12388,#12390,#796,.T.);
#15630=EDGE_CURVE('',#12391,#12392,#7569,.T.);
#15631=EDGE_CURVE('',#12391,#12387,#797,.T.);
#15632=EDGE_CURVE('',#12392,#12388,#798,.T.);
#15633=EDGE_CURVE('',#12393,#12394,#7570,.T.);
#15634=EDGE_CURVE('',#12393,#12391,#799,.T.);
#15635=EDGE_CURVE('',#12394,#12392,#800,.T.);
#15636=EDGE_CURVE('',#12395,#12396,#7571,.T.);
#15637=EDGE_CURVE('',#12395,#12393,#801,.T.);
#15638=EDGE_CURVE('',#12396,#12394,#802,.T.);
#15639=EDGE_CURVE('',#12397,#12398,#7572,.T.);
#15640=EDGE_CURVE('',#12397,#12399,#7573,.T.);
#15641=EDGE_CURVE('',#12400,#12399,#7574,.T.);
#15642=EDGE_CURVE('',#12398,#12400,#271,.T.);
#15643=EDGE_CURVE('',#12400,#12401,#272,.T.);
#15644=EDGE_CURVE('',#12399,#12402,#7575,.T.);
#15645=EDGE_CURVE('',#12401,#12402,#7576,.T.);
#15646=EDGE_CURVE('',#12397,#12402,#2319,.T.);
#15647=EDGE_CURVE('',#12403,#12404,#7577,.T.);
#15648=EDGE_CURVE('',#12403,#12405,#7578,.T.);
#15649=EDGE_CURVE('',#12406,#12405,#7579,.T.);
#15650=EDGE_CURVE('',#12404,#12406,#273,.T.);
#15651=EDGE_CURVE('',#12406,#12407,#274,.T.);
#15652=EDGE_CURVE('',#12405,#12408,#7580,.T.);
#15653=EDGE_CURVE('',#12407,#12408,#7581,.T.);
#15654=EDGE_CURVE('',#12403,#12408,#2320,.T.);
#15655=EDGE_CURVE('',#12409,#12410,#7582,.T.);
#15656=EDGE_CURVE('',#12409,#12411,#7583,.T.);
#15657=EDGE_CURVE('',#12412,#12411,#7584,.T.);
#15658=EDGE_CURVE('',#12410,#12412,#275,.T.);
#15659=EDGE_CURVE('',#12412,#12413,#276,.T.);
#15660=EDGE_CURVE('',#12411,#12414,#7585,.T.);
#15661=EDGE_CURVE('',#12413,#12414,#7586,.T.);
#15662=EDGE_CURVE('',#12409,#12414,#2321,.T.);
#15663=EDGE_CURVE('',#12415,#12416,#7587,.T.);
#15664=EDGE_CURVE('',#12415,#12417,#7588,.T.);
#15665=EDGE_CURVE('',#12418,#12417,#7589,.T.);
#15666=EDGE_CURVE('',#12416,#12418,#277,.T.);
#15667=EDGE_CURVE('',#12418,#12419,#278,.T.);
#15668=EDGE_CURVE('',#12417,#12420,#7590,.T.);
#15669=EDGE_CURVE('',#12419,#12420,#7591,.T.);
#15670=EDGE_CURVE('',#12415,#12420,#2322,.T.);
#15671=EDGE_CURVE('',#12421,#12422,#7592,.T.);
#15672=EDGE_CURVE('',#12421,#12423,#7593,.T.);
#15673=EDGE_CURVE('',#12424,#12423,#7594,.T.);
#15674=EDGE_CURVE('',#12422,#12424,#279,.T.);
#15675=EDGE_CURVE('',#12424,#12425,#280,.T.);
#15676=EDGE_CURVE('',#12423,#12426,#7595,.T.);
#15677=EDGE_CURVE('',#12425,#12426,#7596,.T.);
#15678=EDGE_CURVE('',#12421,#12426,#2323,.T.);
#15679=EDGE_CURVE('',#12427,#12428,#7597,.T.);
#15680=EDGE_CURVE('',#12427,#12429,#7598,.T.);
#15681=EDGE_CURVE('',#12430,#12429,#7599,.T.);
#15682=EDGE_CURVE('',#12428,#12430,#281,.T.);
#15683=EDGE_CURVE('',#12430,#12431,#282,.T.);
#15684=EDGE_CURVE('',#12429,#12432,#7600,.T.);
#15685=EDGE_CURVE('',#12431,#12432,#7601,.T.);
#15686=EDGE_CURVE('',#12427,#12433,#2324,.T.);
#15687=EDGE_CURVE('',#12433,#12432,#2325,.T.);
#15688=EDGE_CURVE('',#12434,#12435,#7602,.T.);
#15689=EDGE_CURVE('',#12434,#12436,#7603,.T.);
#15690=EDGE_CURVE('',#12437,#12436,#7604,.T.);
#15691=EDGE_CURVE('',#12435,#12437,#283,.T.);
#15692=EDGE_CURVE('',#12437,#12438,#284,.T.);
#15693=EDGE_CURVE('',#12436,#12439,#7605,.T.);
#15694=EDGE_CURVE('',#12438,#12439,#7606,.T.);
#15695=EDGE_CURVE('',#12434,#12439,#2326,.T.);
#15696=EDGE_CURVE('',#12440,#12441,#7607,.T.);
#15697=EDGE_CURVE('',#12440,#12442,#7608,.T.);
#15698=EDGE_CURVE('',#12443,#12442,#7609,.T.);
#15699=EDGE_CURVE('',#12441,#12443,#285,.T.);
#15700=EDGE_CURVE('',#12443,#12444,#286,.T.);
#15701=EDGE_CURVE('',#12442,#12445,#7610,.T.);
#15702=EDGE_CURVE('',#12444,#12445,#7611,.T.);
#15703=EDGE_CURVE('',#12440,#12445,#2327,.T.);
#15704=EDGE_CURVE('',#12446,#12447,#7612,.T.);
#15705=EDGE_CURVE('',#12446,#12448,#7613,.T.);
#15706=EDGE_CURVE('',#12449,#12448,#7614,.T.);
#15707=EDGE_CURVE('',#12447,#12449,#287,.T.);
#15708=EDGE_CURVE('',#12449,#12450,#288,.T.);
#15709=EDGE_CURVE('',#12448,#12451,#7615,.T.);
#15710=EDGE_CURVE('',#12450,#12451,#7616,.T.);
#15711=EDGE_CURVE('',#12446,#12451,#2328,.T.);
#15712=EDGE_CURVE('',#12452,#12453,#7617,.T.);
#15713=EDGE_CURVE('',#12452,#12454,#7618,.T.);
#15714=EDGE_CURVE('',#12455,#12454,#7619,.T.);
#15715=EDGE_CURVE('',#12453,#12455,#289,.T.);
#15716=EDGE_CURVE('',#12455,#12456,#290,.T.);
#15717=EDGE_CURVE('',#12454,#12457,#7620,.T.);
#15718=EDGE_CURVE('',#12456,#12457,#7621,.T.);
#15719=EDGE_CURVE('',#12452,#12457,#2329,.T.);
#15720=EDGE_CURVE('',#12458,#12459,#7622,.T.);
#15721=EDGE_CURVE('',#12458,#12460,#7623,.T.);
#15722=EDGE_CURVE('',#12461,#12460,#7624,.T.);
#15723=EDGE_CURVE('',#12459,#12461,#291,.T.);
#15724=EDGE_CURVE('',#12461,#12462,#292,.T.);
#15725=EDGE_CURVE('',#12460,#12463,#7625,.T.);
#15726=EDGE_CURVE('',#12462,#12463,#7626,.T.);
#15727=EDGE_CURVE('',#12458,#12463,#2330,.T.);
#15728=EDGE_CURVE('',#12464,#12465,#7627,.T.);
#15729=EDGE_CURVE('',#12464,#12466,#7628,.T.);
#15730=EDGE_CURVE('',#12467,#12466,#7629,.T.);
#15731=EDGE_CURVE('',#12465,#12467,#293,.T.);
#15732=EDGE_CURVE('',#12467,#12468,#294,.T.);
#15733=EDGE_CURVE('',#12466,#12469,#7630,.T.);
#15734=EDGE_CURVE('',#12468,#12469,#7631,.T.);
#15735=EDGE_CURVE('',#12464,#12469,#2331,.T.);
#15736=EDGE_CURVE('',#12470,#12471,#7632,.T.);
#15737=EDGE_CURVE('',#12470,#12472,#7633,.T.);
#15738=EDGE_CURVE('',#12473,#12472,#7634,.T.);
#15739=EDGE_CURVE('',#12471,#12473,#295,.T.);
#15740=EDGE_CURVE('',#12473,#12474,#296,.T.);
#15741=EDGE_CURVE('',#12472,#12475,#7635,.T.);
#15742=EDGE_CURVE('',#12474,#12475,#7636,.T.);
#15743=EDGE_CURVE('',#12470,#12475,#2332,.T.);
#15744=EDGE_CURVE('',#12476,#12477,#7637,.T.);
#15745=EDGE_CURVE('',#12476,#12478,#7638,.T.);
#15746=EDGE_CURVE('',#12479,#12478,#7639,.T.);
#15747=EDGE_CURVE('',#12477,#12479,#297,.T.);
#15748=EDGE_CURVE('',#12479,#12480,#298,.T.);
#15749=EDGE_CURVE('',#12478,#12481,#7640,.T.);
#15750=EDGE_CURVE('',#12480,#12481,#7641,.T.);
#15751=EDGE_CURVE('',#12476,#12481,#2333,.T.);
#15752=EDGE_CURVE('',#12482,#12483,#7642,.T.);
#15753=EDGE_CURVE('',#12482,#12484,#7643,.T.);
#15754=EDGE_CURVE('',#12485,#12484,#7644,.T.);
#15755=EDGE_CURVE('',#12483,#12485,#299,.T.);
#15756=EDGE_CURVE('',#12485,#12486,#300,.T.);
#15757=EDGE_CURVE('',#12484,#12487,#7645,.T.);
#15758=EDGE_CURVE('',#12486,#12487,#7646,.T.);
#15759=EDGE_CURVE('',#12482,#12487,#2334,.T.);
#15760=EDGE_CURVE('',#12488,#12489,#7647,.T.);
#15761=EDGE_CURVE('',#12488,#12490,#7648,.T.);
#15762=EDGE_CURVE('',#12491,#12490,#7649,.T.);
#15763=EDGE_CURVE('',#12489,#12491,#301,.T.);
#15764=EDGE_CURVE('',#12491,#12492,#302,.T.);
#15765=EDGE_CURVE('',#12490,#12493,#7650,.T.);
#15766=EDGE_CURVE('',#12492,#12493,#7651,.T.);
#15767=EDGE_CURVE('',#12488,#12493,#2335,.T.);
#15768=EDGE_CURVE('',#12494,#12495,#7652,.T.);
#15769=EDGE_CURVE('',#12494,#12496,#7653,.T.);
#15770=EDGE_CURVE('',#12497,#12496,#7654,.T.);
#15771=EDGE_CURVE('',#12495,#12497,#303,.T.);
#15772=EDGE_CURVE('',#12497,#12498,#304,.T.);
#15773=EDGE_CURVE('',#12496,#12499,#7655,.T.);
#15774=EDGE_CURVE('',#12498,#12499,#7656,.T.);
#15775=EDGE_CURVE('',#12494,#12499,#2336,.T.);
#15776=EDGE_CURVE('',#12500,#12501,#7657,.T.);
#15777=EDGE_CURVE('',#12500,#12502,#7658,.T.);
#15778=EDGE_CURVE('',#12503,#12502,#7659,.T.);
#15779=EDGE_CURVE('',#12501,#12503,#305,.T.);
#15780=EDGE_CURVE('',#12503,#12504,#306,.T.);
#15781=EDGE_CURVE('',#12502,#12505,#7660,.T.);
#15782=EDGE_CURVE('',#12504,#12505,#7661,.T.);
#15783=EDGE_CURVE('',#12500,#12505,#2337,.T.);
#15784=EDGE_CURVE('',#12506,#12507,#7662,.T.);
#15785=EDGE_CURVE('',#12506,#12508,#7663,.T.);
#15786=EDGE_CURVE('',#12509,#12508,#7664,.T.);
#15787=EDGE_CURVE('',#12507,#12509,#307,.T.);
#15788=EDGE_CURVE('',#12509,#12510,#308,.T.);
#15789=EDGE_CURVE('',#12508,#12511,#7665,.T.);
#15790=EDGE_CURVE('',#12510,#12511,#7666,.T.);
#15791=EDGE_CURVE('',#12506,#12511,#2338,.T.);
#15792=EDGE_CURVE('',#12512,#12513,#7667,.T.);
#15793=EDGE_CURVE('',#12512,#12514,#7668,.T.);
#15794=EDGE_CURVE('',#12515,#12514,#7669,.T.);
#15795=EDGE_CURVE('',#12513,#12515,#309,.T.);
#15796=EDGE_CURVE('',#12515,#12516,#310,.T.);
#15797=EDGE_CURVE('',#12514,#12517,#7670,.T.);
#15798=EDGE_CURVE('',#12516,#12517,#7671,.T.);
#15799=EDGE_CURVE('',#12512,#12517,#2339,.T.);
#15800=EDGE_CURVE('',#12518,#12519,#7672,.T.);
#15801=EDGE_CURVE('',#12518,#12520,#7673,.T.);
#15802=EDGE_CURVE('',#12521,#12520,#7674,.T.);
#15803=EDGE_CURVE('',#12519,#12521,#311,.T.);
#15804=EDGE_CURVE('',#12521,#12522,#312,.T.);
#15805=EDGE_CURVE('',#12520,#12523,#7675,.T.);
#15806=EDGE_CURVE('',#12522,#12523,#7676,.T.);
#15807=EDGE_CURVE('',#12518,#12523,#2340,.T.);
#15808=EDGE_CURVE('',#12524,#12525,#7677,.T.);
#15809=EDGE_CURVE('',#12524,#12526,#7678,.T.);
#15810=EDGE_CURVE('',#12527,#12526,#7679,.T.);
#15811=EDGE_CURVE('',#12525,#12527,#313,.T.);
#15812=EDGE_CURVE('',#12527,#12528,#314,.T.);
#15813=EDGE_CURVE('',#12526,#12529,#7680,.T.);
#15814=EDGE_CURVE('',#12528,#12529,#7681,.T.);
#15815=EDGE_CURVE('',#12524,#12529,#2341,.T.);
#15816=EDGE_CURVE('',#12530,#12531,#7682,.T.);
#15817=EDGE_CURVE('',#12530,#12532,#7683,.T.);
#15818=EDGE_CURVE('',#12533,#12532,#7684,.T.);
#15819=EDGE_CURVE('',#12531,#12533,#315,.T.);
#15820=EDGE_CURVE('',#12533,#12534,#316,.T.);
#15821=EDGE_CURVE('',#12532,#12535,#7685,.T.);
#15822=EDGE_CURVE('',#12534,#12535,#7686,.T.);
#15823=EDGE_CURVE('',#12530,#12535,#2342,.T.);
#15824=EDGE_CURVE('',#12536,#12537,#7687,.T.);
#15825=EDGE_CURVE('',#12536,#12538,#7688,.T.);
#15826=EDGE_CURVE('',#12539,#12538,#7689,.T.);
#15827=EDGE_CURVE('',#12537,#12539,#317,.T.);
#15828=EDGE_CURVE('',#12539,#12540,#318,.T.);
#15829=EDGE_CURVE('',#12538,#12541,#7690,.T.);
#15830=EDGE_CURVE('',#12540,#12541,#7691,.T.);
#15831=EDGE_CURVE('',#12536,#12541,#2343,.T.);
#15832=EDGE_CURVE('',#12542,#12542,#2344,.T.);
#15833=EDGE_CURVE('',#12542,#12430,#7692,.T.);
#15834=EDGE_CURVE('',#12431,#12507,#2345,.T.);
#15835=EDGE_CURVE('',#12510,#12422,#2346,.T.);
#15836=EDGE_CURVE('',#12425,#12513,#2347,.T.);
#15837=EDGE_CURVE('',#12516,#12416,#2348,.T.);
#15838=EDGE_CURVE('',#12419,#12519,#2349,.T.);
#15839=EDGE_CURVE('',#12522,#12410,#2350,.T.);
#15840=EDGE_CURVE('',#12413,#12525,#2351,.T.);
#15841=EDGE_CURVE('',#12528,#12404,#2352,.T.);
#15842=EDGE_CURVE('',#12407,#12531,#2353,.T.);
#15843=EDGE_CURVE('',#12534,#12398,#2354,.T.);
#15844=EDGE_CURVE('',#12401,#12537,#2355,.T.);
#15845=EDGE_CURVE('',#12540,#12501,#2356,.T.);
#15846=EDGE_CURVE('',#12504,#12465,#2357,.T.);
#15847=EDGE_CURVE('',#12468,#12471,#2358,.T.);
#15848=EDGE_CURVE('',#12474,#12459,#2359,.T.);
#15849=EDGE_CURVE('',#12462,#12477,#2360,.T.);
#15850=EDGE_CURVE('',#12480,#12453,#2361,.T.);
#15851=EDGE_CURVE('',#12456,#12483,#2362,.T.);
#15852=EDGE_CURVE('',#12486,#12447,#2363,.T.);
#15853=EDGE_CURVE('',#12450,#12489,#2364,.T.);
#15854=EDGE_CURVE('',#12492,#12441,#2365,.T.);
#15855=EDGE_CURVE('',#12444,#12495,#2366,.T.);
#15856=EDGE_CURVE('',#12498,#12435,#2367,.T.);
#15857=EDGE_CURVE('',#12438,#12428,#2368,.T.);
#15858=EDGE_CURVE('',#12541,#12500,#2369,.T.);
#15859=EDGE_CURVE('',#12469,#12470,#2370,.T.);
#15860=EDGE_CURVE('',#12505,#12464,#2371,.T.);
#15861=EDGE_CURVE('',#12463,#12476,#2372,.T.);
#15862=EDGE_CURVE('',#12475,#12458,#2373,.T.);
#15863=EDGE_CURVE('',#12457,#12482,#2374,.T.);
#15864=EDGE_CURVE('',#12481,#12452,#2375,.T.);
#15865=EDGE_CURVE('',#12451,#12488,#2376,.T.);
#15866=EDGE_CURVE('',#12487,#12446,#2377,.T.);
#15867=EDGE_CURVE('',#12445,#12494,#2378,.T.);
#15868=EDGE_CURVE('',#12493,#12440,#2379,.T.);
#15869=EDGE_CURVE('',#12499,#12434,#2380,.T.);
#15870=EDGE_CURVE('',#12432,#12506,#2381,.T.);
#15871=EDGE_CURVE('',#12439,#12427,#2382,.T.);
#15872=EDGE_CURVE('',#12426,#12512,#2383,.T.);
#15873=EDGE_CURVE('',#12511,#12421,#2384,.T.);
#15874=EDGE_CURVE('',#12420,#12518,#2385,.T.);
#15875=EDGE_CURVE('',#12517,#12415,#2386,.T.);
#15876=EDGE_CURVE('',#12414,#12524,#2387,.T.);
#15877=EDGE_CURVE('',#12523,#12409,#2388,.T.);
#15878=EDGE_CURVE('',#12408,#12530,#2389,.T.);
#15879=EDGE_CURVE('',#12529,#12403,#2390,.T.);
#15880=EDGE_CURVE('',#12402,#12536,#2391,.T.);
#15881=EDGE_CURVE('',#12543,#12390,#803,.T.);
#15882=EDGE_CURVE('',#12385,#12543,#804,.T.);
#15883=EDGE_CURVE('',#12544,#12377,#805,.T.);
#15884=EDGE_CURVE('',#12544,#12396,#806,.T.);
#15885=EDGE_CURVE('',#12545,#12544,#2392,.T.);
#15886=EDGE_CURVE('',#12545,#12395,#807,.T.);
#15887=EDGE_CURVE('',#12389,#12386,#808,.T.);
#15888=EDGE_CURVE('',#12376,#12545,#809,.T.);
#15889=EDGE_CURVE('',#12384,#12543,#2393,.T.);
#15890=EDGE_CURVE('',#12546,#12546,#2394,.T.);
#15891=EDGE_CURVE('',#12547,#12547,#2395,.T.);
#15892=EDGE_CURVE('',#12547,#12546,#7693,.T.);
#15893=EDGE_CURVE('',#12548,#12548,#2396,.T.);
#15894=EDGE_CURVE('',#12548,#12547,#7694,.T.);
#15895=EDGE_CURVE('',#12549,#12549,#2397,.T.);
#15896=EDGE_CURVE('',#12549,#12548,#7695,.T.);
#15897=EDGE_CURVE('',#12550,#12550,#2398,.T.);
#15898=EDGE_CURVE('',#12535,#12397,#2399,.T.);
#15899=EDGE_CURVE('',#12433,#12550,#7696,.T.);
#21451=ORIENTED_EDGE('',*,*,#15609,.F.);
#21452=ORIENTED_EDGE('',*,*,#15610,.T.);
#21453=ORIENTED_EDGE('',*,*,#15611,.T.);
#21454=ORIENTED_EDGE('',*,*,#15612,.T.);
#21455=ORIENTED_EDGE('',*,*,#15613,.F.);
#21456=ORIENTED_EDGE('',*,*,#15614,.T.);
#21457=ORIENTED_EDGE('',*,*,#15609,.T.);
#21458=ORIENTED_EDGE('',*,*,#15615,.T.);
#21459=ORIENTED_EDGE('',*,*,#15616,.F.);
#21460=ORIENTED_EDGE('',*,*,#15617,.T.);
#21461=ORIENTED_EDGE('',*,*,#15613,.T.);
#21462=ORIENTED_EDGE('',*,*,#15618,.T.);
#21463=ORIENTED_EDGE('',*,*,#15619,.F.);
#21464=ORIENTED_EDGE('',*,*,#15620,.T.);
#21465=ORIENTED_EDGE('',*,*,#15616,.T.);
#21466=ORIENTED_EDGE('',*,*,#15621,.T.);
#21467=ORIENTED_EDGE('',*,*,#15622,.F.);
#21468=ORIENTED_EDGE('',*,*,#15623,.F.);
#21469=ORIENTED_EDGE('',*,*,#15624,.T.);
#21470=ORIENTED_EDGE('',*,*,#15619,.T.);
#21471=ORIENTED_EDGE('',*,*,#15625,.T.);
#21472=ORIENTED_EDGE('',*,*,#15626,.F.);
#21473=ORIENTED_EDGE('',*,*,#15627,.T.);
#21474=ORIENTED_EDGE('',*,*,#15628,.F.);
#21475=ORIENTED_EDGE('',*,*,#15629,.F.);
#21476=ORIENTED_EDGE('',*,*,#15630,.F.);
#21477=ORIENTED_EDGE('',*,*,#15631,.T.);
#21478=ORIENTED_EDGE('',*,*,#15626,.T.);
#21479=ORIENTED_EDGE('',*,*,#15632,.F.);
#21480=ORIENTED_EDGE('',*,*,#15633,.F.);
#21481=ORIENTED_EDGE('',*,*,#15634,.T.);
#21482=ORIENTED_EDGE('',*,*,#15630,.T.);
#21483=ORIENTED_EDGE('',*,*,#15635,.F.);
#21484=ORIENTED_EDGE('',*,*,#15636,.F.);
#21485=ORIENTED_EDGE('',*,*,#15637,.T.);
#21486=ORIENTED_EDGE('',*,*,#15633,.T.);
#21487=ORIENTED_EDGE('',*,*,#15638,.F.);
#21488=ORIENTED_EDGE('',*,*,#15639,.F.);
#21489=ORIENTED_EDGE('',*,*,#15640,.T.);
#21490=ORIENTED_EDGE('',*,*,#15641,.F.);
#21491=ORIENTED_EDGE('',*,*,#15642,.F.);
#21492=ORIENTED_EDGE('',*,*,#15643,.F.);
#21493=ORIENTED_EDGE('',*,*,#15641,.T.);
#21494=ORIENTED_EDGE('',*,*,#15644,.T.);
#21495=ORIENTED_EDGE('',*,*,#15645,.F.);
#21496=ORIENTED_EDGE('',*,*,#15646,.T.);
#21497=ORIENTED_EDGE('',*,*,#15644,.F.);
#21498=ORIENTED_EDGE('',*,*,#15640,.F.);
#21499=ORIENTED_EDGE('',*,*,#15647,.F.);
#21500=ORIENTED_EDGE('',*,*,#15648,.T.);
#21501=ORIENTED_EDGE('',*,*,#15649,.F.);
#21502=ORIENTED_EDGE('',*,*,#15650,.F.);
#21503=ORIENTED_EDGE('',*,*,#15651,.F.);
#21504=ORIENTED_EDGE('',*,*,#15649,.T.);
#21505=ORIENTED_EDGE('',*,*,#15652,.T.);
#21506=ORIENTED_EDGE('',*,*,#15653,.F.);
#21507=ORIENTED_EDGE('',*,*,#15654,.T.);
#21508=ORIENTED_EDGE('',*,*,#15652,.F.);
#21509=ORIENTED_EDGE('',*,*,#15648,.F.);
#21510=ORIENTED_EDGE('',*,*,#15655,.F.);
#21511=ORIENTED_EDGE('',*,*,#15656,.T.);
#21512=ORIENTED_EDGE('',*,*,#15657,.F.);
#21513=ORIENTED_EDGE('',*,*,#15658,.F.);
#21514=ORIENTED_EDGE('',*,*,#15659,.F.);
#21515=ORIENTED_EDGE('',*,*,#15657,.T.);
#21516=ORIENTED_EDGE('',*,*,#15660,.T.);
#21517=ORIENTED_EDGE('',*,*,#15661,.F.);
#21518=ORIENTED_EDGE('',*,*,#15662,.T.);
#21519=ORIENTED_EDGE('',*,*,#15660,.F.);
#21520=ORIENTED_EDGE('',*,*,#15656,.F.);
#21521=ORIENTED_EDGE('',*,*,#15663,.F.);
#21522=ORIENTED_EDGE('',*,*,#15664,.T.);
#21523=ORIENTED_EDGE('',*,*,#15665,.F.);
#21524=ORIENTED_EDGE('',*,*,#15666,.F.);
#21525=ORIENTED_EDGE('',*,*,#15667,.F.);
#21526=ORIENTED_EDGE('',*,*,#15665,.T.);
#21527=ORIENTED_EDGE('',*,*,#15668,.T.);
#21528=ORIENTED_EDGE('',*,*,#15669,.F.);
#21529=ORIENTED_EDGE('',*,*,#15670,.T.);
#21530=ORIENTED_EDGE('',*,*,#15668,.F.);
#21531=ORIENTED_EDGE('',*,*,#15664,.F.);
#21532=ORIENTED_EDGE('',*,*,#15671,.F.);
#21533=ORIENTED_EDGE('',*,*,#15672,.T.);
#21534=ORIENTED_EDGE('',*,*,#15673,.F.);
#21535=ORIENTED_EDGE('',*,*,#15674,.F.);
#21536=ORIENTED_EDGE('',*,*,#15675,.F.);
#21537=ORIENTED_EDGE('',*,*,#15673,.T.);
#21538=ORIENTED_EDGE('',*,*,#15676,.T.);
#21539=ORIENTED_EDGE('',*,*,#15677,.F.);
#21540=ORIENTED_EDGE('',*,*,#15678,.T.);
#21541=ORIENTED_EDGE('',*,*,#15676,.F.);
#21542=ORIENTED_EDGE('',*,*,#15672,.F.);
#21543=ORIENTED_EDGE('',*,*,#15679,.F.);
#21544=ORIENTED_EDGE('',*,*,#15680,.T.);
#21545=ORIENTED_EDGE('',*,*,#15681,.F.);
#21546=ORIENTED_EDGE('',*,*,#15682,.F.);
#21547=ORIENTED_EDGE('',*,*,#15683,.F.);
#21548=ORIENTED_EDGE('',*,*,#15681,.T.);
#21549=ORIENTED_EDGE('',*,*,#15684,.T.);
#21550=ORIENTED_EDGE('',*,*,#15685,.F.);
#21551=ORIENTED_EDGE('',*,*,#15686,.T.);
#21552=ORIENTED_EDGE('',*,*,#15687,.T.);
#21553=ORIENTED_EDGE('',*,*,#15684,.F.);
#21554=ORIENTED_EDGE('',*,*,#15680,.F.);
#21555=ORIENTED_EDGE('',*,*,#15688,.F.);
#21556=ORIENTED_EDGE('',*,*,#15689,.T.);
#21557=ORIENTED_EDGE('',*,*,#15690,.F.);
#21558=ORIENTED_EDGE('',*,*,#15691,.F.);
#21559=ORIENTED_EDGE('',*,*,#15692,.F.);
#21560=ORIENTED_EDGE('',*,*,#15690,.T.);
#21561=ORIENTED_EDGE('',*,*,#15693,.T.);
#21562=ORIENTED_EDGE('',*,*,#15694,.F.);
#21563=ORIENTED_EDGE('',*,*,#15695,.T.);
#21564=ORIENTED_EDGE('',*,*,#15693,.F.);
#21565=ORIENTED_EDGE('',*,*,#15689,.F.);
#21566=ORIENTED_EDGE('',*,*,#15696,.F.);
#21567=ORIENTED_EDGE('',*,*,#15697,.T.);
#21568=ORIENTED_EDGE('',*,*,#15698,.F.);
#21569=ORIENTED_EDGE('',*,*,#15699,.F.);
#21570=ORIENTED_EDGE('',*,*,#15700,.F.);
#21571=ORIENTED_EDGE('',*,*,#15698,.T.);
#21572=ORIENTED_EDGE('',*,*,#15701,.T.);
#21573=ORIENTED_EDGE('',*,*,#15702,.F.);
#21574=ORIENTED_EDGE('',*,*,#15703,.T.);
#21575=ORIENTED_EDGE('',*,*,#15701,.F.);
#21576=ORIENTED_EDGE('',*,*,#15697,.F.);
#21577=ORIENTED_EDGE('',*,*,#15704,.F.);
#21578=ORIENTED_EDGE('',*,*,#15705,.T.);
#21579=ORIENTED_EDGE('',*,*,#15706,.F.);
#21580=ORIENTED_EDGE('',*,*,#15707,.F.);
#21581=ORIENTED_EDGE('',*,*,#15708,.F.);
#21582=ORIENTED_EDGE('',*,*,#15706,.T.);
#21583=ORIENTED_EDGE('',*,*,#15709,.T.);
#21584=ORIENTED_EDGE('',*,*,#15710,.F.);
#21585=ORIENTED_EDGE('',*,*,#15711,.T.);
#21586=ORIENTED_EDGE('',*,*,#15709,.F.);
#21587=ORIENTED_EDGE('',*,*,#15705,.F.);
#21588=ORIENTED_EDGE('',*,*,#15712,.F.);
#21589=ORIENTED_EDGE('',*,*,#15713,.T.);
#21590=ORIENTED_EDGE('',*,*,#15714,.F.);
#21591=ORIENTED_EDGE('',*,*,#15715,.F.);
#21592=ORIENTED_EDGE('',*,*,#15716,.F.);
#21593=ORIENTED_EDGE('',*,*,#15714,.T.);
#21594=ORIENTED_EDGE('',*,*,#15717,.T.);
#21595=ORIENTED_EDGE('',*,*,#15718,.F.);
#21596=ORIENTED_EDGE('',*,*,#15719,.T.);
#21597=ORIENTED_EDGE('',*,*,#15717,.F.);
#21598=ORIENTED_EDGE('',*,*,#15713,.F.);
#21599=ORIENTED_EDGE('',*,*,#15720,.F.);
#21600=ORIENTED_EDGE('',*,*,#15721,.T.);
#21601=ORIENTED_EDGE('',*,*,#15722,.F.);
#21602=ORIENTED_EDGE('',*,*,#15723,.F.);
#21603=ORIENTED_EDGE('',*,*,#15724,.F.);
#21604=ORIENTED_EDGE('',*,*,#15722,.T.);
#21605=ORIENTED_EDGE('',*,*,#15725,.T.);
#21606=ORIENTED_EDGE('',*,*,#15726,.F.);
#21607=ORIENTED_EDGE('',*,*,#15727,.T.);
#21608=ORIENTED_EDGE('',*,*,#15725,.F.);
#21609=ORIENTED_EDGE('',*,*,#15721,.F.);
#21610=ORIENTED_EDGE('',*,*,#15728,.F.);
#21611=ORIENTED_EDGE('',*,*,#15729,.T.);
#21612=ORIENTED_EDGE('',*,*,#15730,.F.);
#21613=ORIENTED_EDGE('',*,*,#15731,.F.);
#21614=ORIENTED_EDGE('',*,*,#15732,.F.);
#21615=ORIENTED_EDGE('',*,*,#15730,.T.);
#21616=ORIENTED_EDGE('',*,*,#15733,.T.);
#21617=ORIENTED_EDGE('',*,*,#15734,.F.);
#21618=ORIENTED_EDGE('',*,*,#15735,.T.);
#21619=ORIENTED_EDGE('',*,*,#15733,.F.);
#21620=ORIENTED_EDGE('',*,*,#15729,.F.);
#21621=ORIENTED_EDGE('',*,*,#15736,.F.);
#21622=ORIENTED_EDGE('',*,*,#15737,.T.);
#21623=ORIENTED_EDGE('',*,*,#15738,.F.);
#21624=ORIENTED_EDGE('',*,*,#15739,.F.);
#21625=ORIENTED_EDGE('',*,*,#15740,.F.);
#21626=ORIENTED_EDGE('',*,*,#15738,.T.);
#21627=ORIENTED_EDGE('',*,*,#15741,.T.);
#21628=ORIENTED_EDGE('',*,*,#15742,.F.);
#21629=ORIENTED_EDGE('',*,*,#15743,.T.);
#21630=ORIENTED_EDGE('',*,*,#15741,.F.);
#21631=ORIENTED_EDGE('',*,*,#15737,.F.);
#21632=ORIENTED_EDGE('',*,*,#15744,.F.);
#21633=ORIENTED_EDGE('',*,*,#15745,.T.);
#21634=ORIENTED_EDGE('',*,*,#15746,.F.);
#21635=ORIENTED_EDGE('',*,*,#15747,.F.);
#21636=ORIENTED_EDGE('',*,*,#15748,.F.);
#21637=ORIENTED_EDGE('',*,*,#15746,.T.);
#21638=ORIENTED_EDGE('',*,*,#15749,.T.);
#21639=ORIENTED_EDGE('',*,*,#15750,.F.);
#21640=ORIENTED_EDGE('',*,*,#15751,.T.);
#21641=ORIENTED_EDGE('',*,*,#15749,.F.);
#21642=ORIENTED_EDGE('',*,*,#15745,.F.);
#21643=ORIENTED_EDGE('',*,*,#15752,.F.);
#21644=ORIENTED_EDGE('',*,*,#15753,.T.);
#21645=ORIENTED_EDGE('',*,*,#15754,.F.);
#21646=ORIENTED_EDGE('',*,*,#15755,.F.);
#21647=ORIENTED_EDGE('',*,*,#15756,.F.);
#21648=ORIENTED_EDGE('',*,*,#15754,.T.);
#21649=ORIENTED_EDGE('',*,*,#15757,.T.);
#21650=ORIENTED_EDGE('',*,*,#15758,.F.);
#21651=ORIENTED_EDGE('',*,*,#15759,.T.);
#21652=ORIENTED_EDGE('',*,*,#15757,.F.);
#21653=ORIENTED_EDGE('',*,*,#15753,.F.);
#21654=ORIENTED_EDGE('',*,*,#15760,.F.);
#21655=ORIENTED_EDGE('',*,*,#15761,.T.);
#21656=ORIENTED_EDGE('',*,*,#15762,.F.);
#21657=ORIENTED_EDGE('',*,*,#15763,.F.);
#21658=ORIENTED_EDGE('',*,*,#15764,.F.);
#21659=ORIENTED_EDGE('',*,*,#15762,.T.);
#21660=ORIENTED_EDGE('',*,*,#15765,.T.);
#21661=ORIENTED_EDGE('',*,*,#15766,.F.);
#21662=ORIENTED_EDGE('',*,*,#15767,.T.);
#21663=ORIENTED_EDGE('',*,*,#15765,.F.);
#21664=ORIENTED_EDGE('',*,*,#15761,.F.);
#21665=ORIENTED_EDGE('',*,*,#15768,.F.);
#21666=ORIENTED_EDGE('',*,*,#15769,.T.);
#21667=ORIENTED_EDGE('',*,*,#15770,.F.);
#21668=ORIENTED_EDGE('',*,*,#15771,.F.);
#21669=ORIENTED_EDGE('',*,*,#15772,.F.);
#21670=ORIENTED_EDGE('',*,*,#15770,.T.);
#21671=ORIENTED_EDGE('',*,*,#15773,.T.);
#21672=ORIENTED_EDGE('',*,*,#15774,.F.);
#21673=ORIENTED_EDGE('',*,*,#15775,.T.);
#21674=ORIENTED_EDGE('',*,*,#15773,.F.);
#21675=ORIENTED_EDGE('',*,*,#15769,.F.);
#21676=ORIENTED_EDGE('',*,*,#15776,.F.);
#21677=ORIENTED_EDGE('',*,*,#15777,.T.);
#21678=ORIENTED_EDGE('',*,*,#15778,.F.);
#21679=ORIENTED_EDGE('',*,*,#15779,.F.);
#21680=ORIENTED_EDGE('',*,*,#15780,.F.);
#21681=ORIENTED_EDGE('',*,*,#15778,.T.);
#21682=ORIENTED_EDGE('',*,*,#15781,.T.);
#21683=ORIENTED_EDGE('',*,*,#15782,.F.);
#21684=ORIENTED_EDGE('',*,*,#15783,.T.);
#21685=ORIENTED_EDGE('',*,*,#15781,.F.);
#21686=ORIENTED_EDGE('',*,*,#15777,.F.);
#21687=ORIENTED_EDGE('',*,*,#15784,.F.);
#21688=ORIENTED_EDGE('',*,*,#15785,.T.);
#21689=ORIENTED_EDGE('',*,*,#15786,.F.);
#21690=ORIENTED_EDGE('',*,*,#15787,.F.);
#21691=ORIENTED_EDGE('',*,*,#15788,.F.);
#21692=ORIENTED_EDGE('',*,*,#15786,.T.);
#21693=ORIENTED_EDGE('',*,*,#15789,.T.);
#21694=ORIENTED_EDGE('',*,*,#15790,.F.);
#21695=ORIENTED_EDGE('',*,*,#15791,.T.);
#21696=ORIENTED_EDGE('',*,*,#15789,.F.);
#21697=ORIENTED_EDGE('',*,*,#15785,.F.);
#21698=ORIENTED_EDGE('',*,*,#15792,.F.);
#21699=ORIENTED_EDGE('',*,*,#15793,.T.);
#21700=ORIENTED_EDGE('',*,*,#15794,.F.);
#21701=ORIENTED_EDGE('',*,*,#15795,.F.);
#21702=ORIENTED_EDGE('',*,*,#15796,.F.);
#21703=ORIENTED_EDGE('',*,*,#15794,.T.);
#21704=ORIENTED_EDGE('',*,*,#15797,.T.);
#21705=ORIENTED_EDGE('',*,*,#15798,.F.);
#21706=ORIENTED_EDGE('',*,*,#15799,.T.);
#21707=ORIENTED_EDGE('',*,*,#15797,.F.);
#21708=ORIENTED_EDGE('',*,*,#15793,.F.);
#21709=ORIENTED_EDGE('',*,*,#15800,.F.);
#21710=ORIENTED_EDGE('',*,*,#15801,.T.);
#21711=ORIENTED_EDGE('',*,*,#15802,.F.);
#21712=ORIENTED_EDGE('',*,*,#15803,.F.);
#21713=ORIENTED_EDGE('',*,*,#15804,.F.);
#21714=ORIENTED_EDGE('',*,*,#15802,.T.);
#21715=ORIENTED_EDGE('',*,*,#15805,.T.);
#21716=ORIENTED_EDGE('',*,*,#15806,.F.);
#21717=ORIENTED_EDGE('',*,*,#15807,.T.);
#21718=ORIENTED_EDGE('',*,*,#15805,.F.);
#21719=ORIENTED_EDGE('',*,*,#15801,.F.);
#21720=ORIENTED_EDGE('',*,*,#15808,.F.);
#21721=ORIENTED_EDGE('',*,*,#15809,.T.);
#21722=ORIENTED_EDGE('',*,*,#15810,.F.);
#21723=ORIENTED_EDGE('',*,*,#15811,.F.);
#21724=ORIENTED_EDGE('',*,*,#15812,.F.);
#21725=ORIENTED_EDGE('',*,*,#15810,.T.);
#21726=ORIENTED_EDGE('',*,*,#15813,.T.);
#21727=ORIENTED_EDGE('',*,*,#15814,.F.);
#21728=ORIENTED_EDGE('',*,*,#15815,.T.);
#21729=ORIENTED_EDGE('',*,*,#15813,.F.);
#21730=ORIENTED_EDGE('',*,*,#15809,.F.);
#21731=ORIENTED_EDGE('',*,*,#15816,.F.);
#21732=ORIENTED_EDGE('',*,*,#15817,.T.);
#21733=ORIENTED_EDGE('',*,*,#15818,.F.);
#21734=ORIENTED_EDGE('',*,*,#15819,.F.);
#21735=ORIENTED_EDGE('',*,*,#15820,.F.);
#21736=ORIENTED_EDGE('',*,*,#15818,.T.);
#21737=ORIENTED_EDGE('',*,*,#15821,.T.);
#21738=ORIENTED_EDGE('',*,*,#15822,.F.);
#21739=ORIENTED_EDGE('',*,*,#15823,.T.);
#21740=ORIENTED_EDGE('',*,*,#15821,.F.);
#21741=ORIENTED_EDGE('',*,*,#15817,.F.);
#21742=ORIENTED_EDGE('',*,*,#15824,.F.);
#21743=ORIENTED_EDGE('',*,*,#15825,.T.);
#21744=ORIENTED_EDGE('',*,*,#15826,.F.);
#21745=ORIENTED_EDGE('',*,*,#15827,.F.);
#21746=ORIENTED_EDGE('',*,*,#15828,.F.);
#21747=ORIENTED_EDGE('',*,*,#15826,.T.);
#21748=ORIENTED_EDGE('',*,*,#15829,.T.);
#21749=ORIENTED_EDGE('',*,*,#15830,.F.);
#21750=ORIENTED_EDGE('',*,*,#15831,.T.);
#21751=ORIENTED_EDGE('',*,*,#15829,.F.);
#21752=ORIENTED_EDGE('',*,*,#15825,.F.);
#21753=ORIENTED_EDGE('',*,*,#15832,.F.);
#21754=ORIENTED_EDGE('',*,*,#15833,.T.);
#21755=ORIENTED_EDGE('',*,*,#15683,.T.);
#21756=ORIENTED_EDGE('',*,*,#15834,.T.);
#21757=ORIENTED_EDGE('',*,*,#15787,.T.);
#21758=ORIENTED_EDGE('',*,*,#15788,.T.);
#21759=ORIENTED_EDGE('',*,*,#15835,.T.);
#21760=ORIENTED_EDGE('',*,*,#15674,.T.);
#21761=ORIENTED_EDGE('',*,*,#15675,.T.);
#21762=ORIENTED_EDGE('',*,*,#15836,.T.);
#21763=ORIENTED_EDGE('',*,*,#15795,.T.);
#21764=ORIENTED_EDGE('',*,*,#15796,.T.);
#21765=ORIENTED_EDGE('',*,*,#15837,.T.);
#21766=ORIENTED_EDGE('',*,*,#15666,.T.);
#21767=ORIENTED_EDGE('',*,*,#15667,.T.);
#21768=ORIENTED_EDGE('',*,*,#15838,.T.);
#21769=ORIENTED_EDGE('',*,*,#15803,.T.);
#21770=ORIENTED_EDGE('',*,*,#15804,.T.);
#21771=ORIENTED_EDGE('',*,*,#15839,.T.);
#21772=ORIENTED_EDGE('',*,*,#15658,.T.);
#21773=ORIENTED_EDGE('',*,*,#15659,.T.);
#21774=ORIENTED_EDGE('',*,*,#15840,.T.);
#21775=ORIENTED_EDGE('',*,*,#15811,.T.);
#21776=ORIENTED_EDGE('',*,*,#15812,.T.);
#21777=ORIENTED_EDGE('',*,*,#15841,.T.);
#21778=ORIENTED_EDGE('',*,*,#15650,.T.);
#21779=ORIENTED_EDGE('',*,*,#15651,.T.);
#21780=ORIENTED_EDGE('',*,*,#15842,.T.);
#21781=ORIENTED_EDGE('',*,*,#15819,.T.);
#21782=ORIENTED_EDGE('',*,*,#15820,.T.);
#21783=ORIENTED_EDGE('',*,*,#15843,.T.);
#21784=ORIENTED_EDGE('',*,*,#15642,.T.);
#21785=ORIENTED_EDGE('',*,*,#15643,.T.);
#21786=ORIENTED_EDGE('',*,*,#15844,.T.);
#21787=ORIENTED_EDGE('',*,*,#15827,.T.);
#21788=ORIENTED_EDGE('',*,*,#15828,.T.);
#21789=ORIENTED_EDGE('',*,*,#15845,.T.);
#21790=ORIENTED_EDGE('',*,*,#15779,.T.);
#21791=ORIENTED_EDGE('',*,*,#15780,.T.);
#21792=ORIENTED_EDGE('',*,*,#15846,.T.);
#21793=ORIENTED_EDGE('',*,*,#15731,.T.);
#21794=ORIENTED_EDGE('',*,*,#15732,.T.);
#21795=ORIENTED_EDGE('',*,*,#15847,.T.);
#21796=ORIENTED_EDGE('',*,*,#15739,.T.);
#21797=ORIENTED_EDGE('',*,*,#15740,.T.);
#21798=ORIENTED_EDGE('',*,*,#15848,.T.);
#21799=ORIENTED_EDGE('',*,*,#15723,.T.);
#21800=ORIENTED_EDGE('',*,*,#15724,.T.);
#21801=ORIENTED_EDGE('',*,*,#15849,.T.);
#21802=ORIENTED_EDGE('',*,*,#15747,.T.);
#21803=ORIENTED_EDGE('',*,*,#15748,.T.);
#21804=ORIENTED_EDGE('',*,*,#15850,.T.);
#21805=ORIENTED_EDGE('',*,*,#15715,.T.);
#21806=ORIENTED_EDGE('',*,*,#15716,.T.);
#21807=ORIENTED_EDGE('',*,*,#15851,.T.);
#21808=ORIENTED_EDGE('',*,*,#15755,.T.);
#21809=ORIENTED_EDGE('',*,*,#15756,.T.);
#21810=ORIENTED_EDGE('',*,*,#15852,.T.);
#21811=ORIENTED_EDGE('',*,*,#15707,.T.);
#21812=ORIENTED_EDGE('',*,*,#15708,.T.);
#21813=ORIENTED_EDGE('',*,*,#15853,.T.);
#21814=ORIENTED_EDGE('',*,*,#15763,.T.);
#21815=ORIENTED_EDGE('',*,*,#15764,.T.);
#21816=ORIENTED_EDGE('',*,*,#15854,.T.);
#21817=ORIENTED_EDGE('',*,*,#15699,.T.);
#21818=ORIENTED_EDGE('',*,*,#15700,.T.);
#21819=ORIENTED_EDGE('',*,*,#15855,.T.);
#21820=ORIENTED_EDGE('',*,*,#15771,.T.);
#21821=ORIENTED_EDGE('',*,*,#15772,.T.);
#21822=ORIENTED_EDGE('',*,*,#15856,.T.);
#21823=ORIENTED_EDGE('',*,*,#15691,.T.);
#21824=ORIENTED_EDGE('',*,*,#15692,.T.);
#21825=ORIENTED_EDGE('',*,*,#15857,.T.);
#21826=ORIENTED_EDGE('',*,*,#15682,.T.);
#21827=ORIENTED_EDGE('',*,*,#15833,.F.);
#21828=ORIENTED_EDGE('',*,*,#15776,.T.);
#21829=ORIENTED_EDGE('',*,*,#15845,.F.);
#21830=ORIENTED_EDGE('',*,*,#15830,.T.);
#21831=ORIENTED_EDGE('',*,*,#15858,.T.);
#21832=ORIENTED_EDGE('',*,*,#15734,.T.);
#21833=ORIENTED_EDGE('',*,*,#15859,.T.);
#21834=ORIENTED_EDGE('',*,*,#15736,.T.);
#21835=ORIENTED_EDGE('',*,*,#15847,.F.);
#21836=ORIENTED_EDGE('',*,*,#15728,.T.);
#21837=ORIENTED_EDGE('',*,*,#15846,.F.);
#21838=ORIENTED_EDGE('',*,*,#15782,.T.);
#21839=ORIENTED_EDGE('',*,*,#15860,.T.);
#21840=ORIENTED_EDGE('',*,*,#15726,.T.);
#21841=ORIENTED_EDGE('',*,*,#15861,.T.);
#21842=ORIENTED_EDGE('',*,*,#15744,.T.);
#21843=ORIENTED_EDGE('',*,*,#15849,.F.);
#21844=ORIENTED_EDGE('',*,*,#15720,.T.);
#21845=ORIENTED_EDGE('',*,*,#15848,.F.);
#21846=ORIENTED_EDGE('',*,*,#15742,.T.);
#21847=ORIENTED_EDGE('',*,*,#15862,.T.);
#21848=ORIENTED_EDGE('',*,*,#15718,.T.);
#21849=ORIENTED_EDGE('',*,*,#15863,.T.);
#21850=ORIENTED_EDGE('',*,*,#15752,.T.);
#21851=ORIENTED_EDGE('',*,*,#15851,.F.);
#21852=ORIENTED_EDGE('',*,*,#15712,.T.);
#21853=ORIENTED_EDGE('',*,*,#15850,.F.);
#21854=ORIENTED_EDGE('',*,*,#15750,.T.);
#21855=ORIENTED_EDGE('',*,*,#15864,.T.);
#21856=ORIENTED_EDGE('',*,*,#15710,.T.);
#21857=ORIENTED_EDGE('',*,*,#15865,.T.);
#21858=ORIENTED_EDGE('',*,*,#15760,.T.);
#21859=ORIENTED_EDGE('',*,*,#15853,.F.);
#21860=ORIENTED_EDGE('',*,*,#15704,.T.);
#21861=ORIENTED_EDGE('',*,*,#15852,.F.);
#21862=ORIENTED_EDGE('',*,*,#15758,.T.);
#21863=ORIENTED_EDGE('',*,*,#15866,.T.);
#21864=ORIENTED_EDGE('',*,*,#15702,.T.);
#21865=ORIENTED_EDGE('',*,*,#15867,.T.);
#21866=ORIENTED_EDGE('',*,*,#15768,.T.);
#21867=ORIENTED_EDGE('',*,*,#15855,.F.);
#21868=ORIENTED_EDGE('',*,*,#15696,.T.);
#21869=ORIENTED_EDGE('',*,*,#15854,.F.);
#21870=ORIENTED_EDGE('',*,*,#15766,.T.);
#21871=ORIENTED_EDGE('',*,*,#15868,.T.);
#21872=ORIENTED_EDGE('',*,*,#15688,.T.);
#21873=ORIENTED_EDGE('',*,*,#15856,.F.);
#21874=ORIENTED_EDGE('',*,*,#15774,.T.);
#21875=ORIENTED_EDGE('',*,*,#15869,.T.);
#21876=ORIENTED_EDGE('',*,*,#15685,.T.);
#21877=ORIENTED_EDGE('',*,*,#15870,.T.);
#21878=ORIENTED_EDGE('',*,*,#15784,.T.);
#21879=ORIENTED_EDGE('',*,*,#15834,.F.);
#21880=ORIENTED_EDGE('',*,*,#15679,.T.);
#21881=ORIENTED_EDGE('',*,*,#15857,.F.);
#21882=ORIENTED_EDGE('',*,*,#15694,.T.);
#21883=ORIENTED_EDGE('',*,*,#15871,.T.);
#21884=ORIENTED_EDGE('',*,*,#15677,.T.);
#21885=ORIENTED_EDGE('',*,*,#15872,.T.);
#21886=ORIENTED_EDGE('',*,*,#15792,.T.);
#21887=ORIENTED_EDGE('',*,*,#15836,.F.);
#21888=ORIENTED_EDGE('',*,*,#15671,.T.);
#21889=ORIENTED_EDGE('',*,*,#15835,.F.);
#21890=ORIENTED_EDGE('',*,*,#15790,.T.);
#21891=ORIENTED_EDGE('',*,*,#15873,.T.);
#21892=ORIENTED_EDGE('',*,*,#15669,.T.);
#21893=ORIENTED_EDGE('',*,*,#15874,.T.);
#21894=ORIENTED_EDGE('',*,*,#15800,.T.);
#21895=ORIENTED_EDGE('',*,*,#15838,.F.);
#21896=ORIENTED_EDGE('',*,*,#15663,.T.);
#21897=ORIENTED_EDGE('',*,*,#15837,.F.);
#21898=ORIENTED_EDGE('',*,*,#15798,.T.);
#21899=ORIENTED_EDGE('',*,*,#15875,.T.);
#21900=ORIENTED_EDGE('',*,*,#15661,.T.);
#21901=ORIENTED_EDGE('',*,*,#15876,.T.);
#21902=ORIENTED_EDGE('',*,*,#15808,.T.);
#21903=ORIENTED_EDGE('',*,*,#15840,.F.);
#21904=ORIENTED_EDGE('',*,*,#15655,.T.);
#21905=ORIENTED_EDGE('',*,*,#15839,.F.);
#21906=ORIENTED_EDGE('',*,*,#15806,.T.);
#21907=ORIENTED_EDGE('',*,*,#15877,.T.);
#21908=ORIENTED_EDGE('',*,*,#15653,.T.);
#21909=ORIENTED_EDGE('',*,*,#15878,.T.);
#21910=ORIENTED_EDGE('',*,*,#15816,.T.);
#21911=ORIENTED_EDGE('',*,*,#15842,.F.);
#21912=ORIENTED_EDGE('',*,*,#15647,.T.);
#21913=ORIENTED_EDGE('',*,*,#15841,.F.);
#21914=ORIENTED_EDGE('',*,*,#15814,.T.);
#21915=ORIENTED_EDGE('',*,*,#15879,.T.);
#21916=ORIENTED_EDGE('',*,*,#15645,.T.);
#21917=ORIENTED_EDGE('',*,*,#15880,.T.);
#21918=ORIENTED_EDGE('',*,*,#15824,.T.);
#21919=ORIENTED_EDGE('',*,*,#15844,.F.);
#21920=ORIENTED_EDGE('',*,*,#15881,.F.);
#21921=ORIENTED_EDGE('',*,*,#15882,.F.);
#21922=ORIENTED_EDGE('',*,*,#15625,.F.);
#21923=ORIENTED_EDGE('',*,*,#15621,.F.);
#21924=ORIENTED_EDGE('',*,*,#15618,.F.);
#21925=ORIENTED_EDGE('',*,*,#15615,.F.);
#21926=ORIENTED_EDGE('',*,*,#15612,.F.);
#21927=ORIENTED_EDGE('',*,*,#15883,.F.);
#21928=ORIENTED_EDGE('',*,*,#15884,.T.);
#21929=ORIENTED_EDGE('',*,*,#15638,.T.);
#21930=ORIENTED_EDGE('',*,*,#15635,.T.);
#21931=ORIENTED_EDGE('',*,*,#15632,.T.);
#21932=ORIENTED_EDGE('',*,*,#15629,.T.);
#21933=ORIENTED_EDGE('',*,*,#15636,.T.);
#21934=ORIENTED_EDGE('',*,*,#15884,.F.);
#21935=ORIENTED_EDGE('',*,*,#15885,.F.);
#21936=ORIENTED_EDGE('',*,*,#15886,.T.);
#21937=ORIENTED_EDGE('',*,*,#15887,.F.);
#21938=ORIENTED_EDGE('',*,*,#15627,.F.);
#21939=ORIENTED_EDGE('',*,*,#15631,.F.);
#21940=ORIENTED_EDGE('',*,*,#15634,.F.);
#21941=ORIENTED_EDGE('',*,*,#15637,.F.);
#21942=ORIENTED_EDGE('',*,*,#15886,.F.);
#21943=ORIENTED_EDGE('',*,*,#15888,.F.);
#21944=ORIENTED_EDGE('',*,*,#15610,.F.);
#21945=ORIENTED_EDGE('',*,*,#15614,.F.);
#21946=ORIENTED_EDGE('',*,*,#15617,.F.);
#21947=ORIENTED_EDGE('',*,*,#15620,.F.);
#21948=ORIENTED_EDGE('',*,*,#15624,.F.);
#21949=ORIENTED_EDGE('',*,*,#15622,.T.);
#21950=ORIENTED_EDGE('',*,*,#15882,.T.);
#21951=ORIENTED_EDGE('',*,*,#15889,.F.);
#21952=ORIENTED_EDGE('',*,*,#15890,.F.);
#21953=ORIENTED_EDGE('',*,*,#15891,.F.);
#21954=ORIENTED_EDGE('',*,*,#15892,.T.);
#21955=ORIENTED_EDGE('',*,*,#15890,.T.);
#21956=ORIENTED_EDGE('',*,*,#15892,.F.);
#21957=ORIENTED_EDGE('',*,*,#15893,.F.);
#21958=ORIENTED_EDGE('',*,*,#15894,.T.);
#21959=ORIENTED_EDGE('',*,*,#15891,.T.);
#21960=ORIENTED_EDGE('',*,*,#15894,.F.);
#21961=ORIENTED_EDGE('',*,*,#15895,.F.);
#21962=ORIENTED_EDGE('',*,*,#15896,.T.);
#21963=ORIENTED_EDGE('',*,*,#15893,.T.);
#21964=ORIENTED_EDGE('',*,*,#15896,.F.);
#21965=ORIENTED_EDGE('',*,*,#15895,.T.);
#21966=ORIENTED_EDGE('',*,*,#15888,.T.);
#21967=ORIENTED_EDGE('',*,*,#15885,.T.);
#21968=ORIENTED_EDGE('',*,*,#15883,.T.);
#21969=ORIENTED_EDGE('',*,*,#15611,.F.);
#21970=ORIENTED_EDGE('',*,*,#15897,.F.);
#21971=ORIENTED_EDGE('',*,*,#15623,.T.);
#21972=ORIENTED_EDGE('',*,*,#15889,.T.);
#21973=ORIENTED_EDGE('',*,*,#15881,.T.);
#21974=ORIENTED_EDGE('',*,*,#15628,.T.);
#21975=ORIENTED_EDGE('',*,*,#15887,.T.);
#21976=ORIENTED_EDGE('',*,*,#15783,.F.);
#21977=ORIENTED_EDGE('',*,*,#15858,.F.);
#21978=ORIENTED_EDGE('',*,*,#15831,.F.);
#21979=ORIENTED_EDGE('',*,*,#15880,.F.);
#21980=ORIENTED_EDGE('',*,*,#15646,.F.);
#21981=ORIENTED_EDGE('',*,*,#15898,.F.);
#21982=ORIENTED_EDGE('',*,*,#15823,.F.);
#21983=ORIENTED_EDGE('',*,*,#15878,.F.);
#21984=ORIENTED_EDGE('',*,*,#15654,.F.);
#21985=ORIENTED_EDGE('',*,*,#15879,.F.);
#21986=ORIENTED_EDGE('',*,*,#15815,.F.);
#21987=ORIENTED_EDGE('',*,*,#15876,.F.);
#21988=ORIENTED_EDGE('',*,*,#15662,.F.);
#21989=ORIENTED_EDGE('',*,*,#15877,.F.);
#21990=ORIENTED_EDGE('',*,*,#15807,.F.);
#21991=ORIENTED_EDGE('',*,*,#15874,.F.);
#21992=ORIENTED_EDGE('',*,*,#15670,.F.);
#21993=ORIENTED_EDGE('',*,*,#15875,.F.);
#21994=ORIENTED_EDGE('',*,*,#15799,.F.);
#21995=ORIENTED_EDGE('',*,*,#15872,.F.);
#21996=ORIENTED_EDGE('',*,*,#15678,.F.);
#21997=ORIENTED_EDGE('',*,*,#15873,.F.);
#21998=ORIENTED_EDGE('',*,*,#15791,.F.);
#21999=ORIENTED_EDGE('',*,*,#15870,.F.);
#22000=ORIENTED_EDGE('',*,*,#15687,.F.);
#22001=ORIENTED_EDGE('',*,*,#15899,.T.);
#22002=ORIENTED_EDGE('',*,*,#15897,.T.);
#22003=ORIENTED_EDGE('',*,*,#15899,.F.);
#22004=ORIENTED_EDGE('',*,*,#15686,.F.);
#22005=ORIENTED_EDGE('',*,*,#15871,.F.);
#22006=ORIENTED_EDGE('',*,*,#15695,.F.);
#22007=ORIENTED_EDGE('',*,*,#15869,.F.);
#22008=ORIENTED_EDGE('',*,*,#15775,.F.);
#22009=ORIENTED_EDGE('',*,*,#15867,.F.);
#22010=ORIENTED_EDGE('',*,*,#15703,.F.);
#22011=ORIENTED_EDGE('',*,*,#15868,.F.);
#22012=ORIENTED_EDGE('',*,*,#15767,.F.);
#22013=ORIENTED_EDGE('',*,*,#15865,.F.);
#22014=ORIENTED_EDGE('',*,*,#15711,.F.);
#22015=ORIENTED_EDGE('',*,*,#15866,.F.);
#22016=ORIENTED_EDGE('',*,*,#15759,.F.);
#22017=ORIENTED_EDGE('',*,*,#15863,.F.);
#22018=ORIENTED_EDGE('',*,*,#15719,.F.);
#22019=ORIENTED_EDGE('',*,*,#15864,.F.);
#22020=ORIENTED_EDGE('',*,*,#15751,.F.);
#22021=ORIENTED_EDGE('',*,*,#15861,.F.);
#22022=ORIENTED_EDGE('',*,*,#15727,.F.);
#22023=ORIENTED_EDGE('',*,*,#15862,.F.);
#22024=ORIENTED_EDGE('',*,*,#15743,.F.);
#22025=ORIENTED_EDGE('',*,*,#15859,.F.);
#22026=ORIENTED_EDGE('',*,*,#15735,.F.);
#22027=ORIENTED_EDGE('',*,*,#15860,.F.);
#22028=ORIENTED_EDGE('',*,*,#15639,.T.);
#22029=ORIENTED_EDGE('',*,*,#15843,.F.);
#22030=ORIENTED_EDGE('',*,*,#15822,.T.);
#22031=ORIENTED_EDGE('',*,*,#15898,.T.);
#22032=ORIENTED_EDGE('',*,*,#15832,.T.);
#26459=PLANE('',#29548);
#26460=PLANE('',#29549);
#26461=PLANE('',#29550);
#26462=PLANE('',#29552);
#26463=PLANE('',#29553);
#26464=PLANE('',#29554);
#26465=PLANE('',#29556);
#26466=PLANE('',#29557);
#26467=PLANE('',#29558);
#26468=PLANE('',#29560);
#26469=PLANE('',#29561);
#26470=PLANE('',#29562);
#26471=PLANE('',#29564);
#26472=PLANE('',#29565);
#26473=PLANE('',#29566);
#26474=PLANE('',#29568);
#26475=PLANE('',#29569);
#26476=PLANE('',#29570);
#26477=PLANE('',#29573);
#26478=PLANE('',#29574);
#26479=PLANE('',#29575);
#26480=PLANE('',#29577);
#26481=PLANE('',#29578);
#26482=PLANE('',#29579);
#26483=PLANE('',#29581);
#26484=PLANE('',#29582);
#26485=PLANE('',#29583);
#26486=PLANE('',#29585);
#26487=PLANE('',#29586);
#26488=PLANE('',#29587);
#26489=PLANE('',#29589);
#26490=PLANE('',#29590);
#26491=PLANE('',#29591);
#26492=PLANE('',#29593);
#26493=PLANE('',#29594);
#26494=PLANE('',#29595);
#26495=PLANE('',#29597);
#26496=PLANE('',#29598);
#26497=PLANE('',#29599);
#26498=PLANE('',#29601);
#26499=PLANE('',#29602);
#26500=PLANE('',#29603);
#26501=PLANE('',#29605);
#26502=PLANE('',#29606);
#26503=PLANE('',#29607);
#26504=PLANE('',#29609);
#26505=PLANE('',#29610);
#26506=PLANE('',#29611);
#26507=PLANE('',#29613);
#26508=PLANE('',#29614);
#26509=PLANE('',#29615);
#26510=PLANE('',#29617);
#26511=PLANE('',#29618);
#26512=PLANE('',#29619);
#26513=PLANE('',#29621);
#26514=PLANE('',#29622);
#26515=PLANE('',#29623);
#26516=PLANE('',#29625);
#26517=PLANE('',#29626);
#26518=PLANE('',#29627);
#26519=PLANE('',#29629);
#26520=PLANE('',#29630);
#26521=PLANE('',#29631);
#26522=PLANE('',#29633);
#26523=PLANE('',#29634);
#26524=PLANE('',#29635);
#26525=PLANE('',#29637);
#26526=PLANE('',#29638);
#26527=PLANE('',#29639);
#26528=PLANE('',#29641);
#26529=PLANE('',#29642);
#26530=PLANE('',#29643);
#26531=PLANE('',#29721);
#26532=PLANE('',#29729);
#26533=PLANE('',#29730);
#26534=PLANE('',#29735);
#27555=ADVANCED_FACE('',(#3647),#1592,.T.);
#27556=ADVANCED_FACE('',(#3648),#1593,.T.);
#27557=ADVANCED_FACE('',(#3649),#1594,.T.);
#27558=ADVANCED_FACE('',(#3650),#1595,.T.);
#27559=ADVANCED_FACE('',(#3651),#1596,.T.);
#27560=ADVANCED_FACE('',(#3652),#1597,.T.);
#27561=ADVANCED_FACE('',(#3653),#1598,.T.);
#27562=ADVANCED_FACE('',(#3654),#1599,.T.);
#27563=ADVANCED_FACE('',(#3655),#1600,.T.);
#27564=ADVANCED_FACE('',(#3656),#26459,.F.);
#27565=ADVANCED_FACE('',(#3657),#26460,.F.);
#27566=ADVANCED_FACE('',(#3658),#26461,.F.);
#27567=ADVANCED_FACE('',(#3659),#26462,.F.);
#27568=ADVANCED_FACE('',(#3660),#26463,.F.);
#27569=ADVANCED_FACE('',(#3661),#26464,.F.);
#27570=ADVANCED_FACE('',(#3662),#26465,.F.);
#27571=ADVANCED_FACE('',(#3663),#26466,.F.);
#27572=ADVANCED_FACE('',(#3664),#26467,.F.);
#27573=ADVANCED_FACE('',(#3665),#26468,.F.);
#27574=ADVANCED_FACE('',(#3666),#26469,.F.);
#27575=ADVANCED_FACE('',(#3667),#26470,.F.);
#27576=ADVANCED_FACE('',(#3668),#26471,.F.);
#27577=ADVANCED_FACE('',(#3669),#26472,.F.);
#27578=ADVANCED_FACE('',(#3670),#26473,.F.);
#27579=ADVANCED_FACE('',(#3671),#26474,.F.);
#27580=ADVANCED_FACE('',(#3672),#26475,.F.);
#27581=ADVANCED_FACE('',(#3673),#26476,.F.);
#27582=ADVANCED_FACE('',(#3674),#26477,.F.);
#27583=ADVANCED_FACE('',(#3675),#26478,.F.);
#27584=ADVANCED_FACE('',(#3676),#26479,.F.);
#27585=ADVANCED_FACE('',(#3677),#26480,.F.);
#27586=ADVANCED_FACE('',(#3678),#26481,.F.);
#27587=ADVANCED_FACE('',(#3679),#26482,.F.);
#27588=ADVANCED_FACE('',(#3680),#26483,.F.);
#27589=ADVANCED_FACE('',(#3681),#26484,.F.);
#27590=ADVANCED_FACE('',(#3682),#26485,.F.);
#27591=ADVANCED_FACE('',(#3683),#26486,.F.);
#27592=ADVANCED_FACE('',(#3684),#26487,.F.);
#27593=ADVANCED_FACE('',(#3685),#26488,.F.);
#27594=ADVANCED_FACE('',(#3686),#26489,.F.);
#27595=ADVANCED_FACE('',(#3687),#26490,.F.);
#27596=ADVANCED_FACE('',(#3688),#26491,.F.);
#27597=ADVANCED_FACE('',(#3689),#26492,.F.);
#27598=ADVANCED_FACE('',(#3690),#26493,.F.);
#27599=ADVANCED_FACE('',(#3691),#26494,.F.);
#27600=ADVANCED_FACE('',(#3692),#26495,.F.);
#27601=ADVANCED_FACE('',(#3693),#26496,.F.);
#27602=ADVANCED_FACE('',(#3694),#26497,.F.);
#27603=ADVANCED_FACE('',(#3695),#26498,.F.);
#27604=ADVANCED_FACE('',(#3696),#26499,.F.);
#27605=ADVANCED_FACE('',(#3697),#26500,.F.);
#27606=ADVANCED_FACE('',(#3698),#26501,.F.);
#27607=ADVANCED_FACE('',(#3699),#26502,.F.);
#27608=ADVANCED_FACE('',(#3700),#26503,.F.);
#27609=ADVANCED_FACE('',(#3701),#26504,.F.);
#27610=ADVANCED_FACE('',(#3702),#26505,.F.);
#27611=ADVANCED_FACE('',(#3703),#26506,.F.);
#27612=ADVANCED_FACE('',(#3704),#26507,.F.);
#27613=ADVANCED_FACE('',(#3705),#26508,.F.);
#27614=ADVANCED_FACE('',(#3706),#26509,.F.);
#27615=ADVANCED_FACE('',(#3707),#26510,.F.);
#27616=ADVANCED_FACE('',(#3708),#26511,.F.);
#27617=ADVANCED_FACE('',(#3709),#26512,.F.);
#27618=ADVANCED_FACE('',(#3710),#26513,.F.);
#27619=ADVANCED_FACE('',(#3711),#26514,.F.);
#27620=ADVANCED_FACE('',(#3712),#26515,.F.);
#27621=ADVANCED_FACE('',(#3713),#26516,.F.);
#27622=ADVANCED_FACE('',(#3714),#26517,.F.);
#27623=ADVANCED_FACE('',(#3715),#26518,.F.);
#27624=ADVANCED_FACE('',(#3716),#26519,.F.);
#27625=ADVANCED_FACE('',(#3717),#26520,.F.);
#27626=ADVANCED_FACE('',(#3718),#26521,.F.);
#27627=ADVANCED_FACE('',(#3719),#26522,.F.);
#27628=ADVANCED_FACE('',(#3720),#26523,.F.);
#27629=ADVANCED_FACE('',(#3721),#26524,.F.);
#27630=ADVANCED_FACE('',(#3722),#26525,.F.);
#27631=ADVANCED_FACE('',(#3723),#26526,.F.);
#27632=ADVANCED_FACE('',(#3724),#26527,.F.);
#27633=ADVANCED_FACE('',(#3725),#26528,.F.);
#27634=ADVANCED_FACE('',(#3726),#26529,.F.);
#27635=ADVANCED_FACE('',(#3727),#26530,.F.);
#27636=ADVANCED_FACE('',(#3728),#2852,.T.);
#27637=ADVANCED_FACE('',(#3729),#1601,.T.);
#27638=ADVANCED_FACE('',(#3730),#1602,.T.);
#27639=ADVANCED_FACE('',(#3731),#1603,.T.);
#27640=ADVANCED_FACE('',(#3732),#1604,.T.);
#27641=ADVANCED_FACE('',(#3733),#1605,.T.);
#27642=ADVANCED_FACE('',(#3734),#1606,.T.);
#27643=ADVANCED_FACE('',(#3735),#1607,.T.);
#27644=ADVANCED_FACE('',(#3736),#1608,.T.);
#27645=ADVANCED_FACE('',(#3737),#1609,.T.);
#27646=ADVANCED_FACE('',(#3738),#1610,.T.);
#27647=ADVANCED_FACE('',(#3739),#1611,.T.);
#27648=ADVANCED_FACE('',(#3740),#1612,.T.);
#27649=ADVANCED_FACE('',(#3741),#1613,.T.);
#27650=ADVANCED_FACE('',(#3742),#1614,.T.);
#27651=ADVANCED_FACE('',(#3743),#1615,.T.);
#27652=ADVANCED_FACE('',(#3744),#1616,.T.);
#27653=ADVANCED_FACE('',(#3745),#1617,.T.);
#27654=ADVANCED_FACE('',(#3746),#1618,.T.);
#27655=ADVANCED_FACE('',(#3747),#1619,.T.);
#27656=ADVANCED_FACE('',(#3748),#1620,.T.);
#27657=ADVANCED_FACE('',(#3749),#1621,.T.);
#27658=ADVANCED_FACE('',(#3750),#1622,.T.);
#27659=ADVANCED_FACE('',(#3751),#1623,.T.);
#27660=ADVANCED_FACE('',(#3752),#1454,.F.);
#27661=ADVANCED_FACE('',(#3753),#1624,.T.);
#27662=ADVANCED_FACE('',(#3754),#1455,.F.);
#27663=ADVANCED_FACE('',(#3755),#1625,.T.);
#27664=ADVANCED_FACE('',(#3756),#26531,.T.);
#27665=ADVANCED_FACE('',(#3757),#2853,.T.);
#27666=ADVANCED_FACE('',(#3758),#1626,.T.);
#27667=ADVANCED_FACE('',(#3759),#2854,.T.);
#27668=ADVANCED_FACE('',(#3760,#1928),#26532,.T.);
#27669=ADVANCED_FACE('',(#3761,#1929),#26533,.T.);
#27670=ADVANCED_FACE('',(#3762),#2855,.T.);
#27671=ADVANCED_FACE('',(#3763),#1627,.T.);
#27672=ADVANCED_FACE('',(#3764),#26534,.T.);
#28464=CLOSED_SHELL('',(#27555,#27556,#27557,#27558,#27559,#27560,#27561,
#27562,#27563,#27564,#27565,#27566,#27567,#27568,#27569,#27570,#27571,#27572,
#27573,#27574,#27575,#27576,#27577,#27578,#27579,#27580,#27581,#27582,#27583,
#27584,#27585,#27586,#27587,#27588,#27589,#27590,#27591,#27592,#27593,#27594,
#27595,#27596,#27597,#27598,#27599,#27600,#27601,#27602,#27603,#27604,#27605,
#27606,#27607,#27608,#27609,#27610,#27611,#27612,#27613,#27614,#27615,#27616,
#27617,#27618,#27619,#27620,#27621,#27622,#27623,#27624,#27625,#27626,#27627,
#27628,#27629,#27630,#27631,#27632,#27633,#27634,#27635,#27636,#27637,#27638,
#27639,#27640,#27641,#27642,#27643,#27644,#27645,#27646,#27647,#27648,#27649,
#27650,#27651,#27652,#27653,#27654,#27655,#27656,#27657,#27658,#27659,#27660,
#27661,#27662,#27663,#27664,#27665,#27666,#27667,#27668,#27669,#27670,#27671,
#27672));
#29535=AXIS2_PLACEMENT_3D('',#44018,#33810,#33811);
#29536=AXIS2_PLACEMENT_3D('',#44019,#33812,#33813);
#29537=AXIS2_PLACEMENT_3D('',#44041,#33815,#33816);
#29538=AXIS2_PLACEMENT_3D('',#44052,#33817,#33818);
#29539=AXIS2_PLACEMENT_3D('',#44142,#33820,#33821);
#29540=AXIS2_PLACEMENT_3D('',#44232,#33823,#33824);
#29541=AXIS2_PLACEMENT_3D('',#44322,#33826,#33827);
#29542=AXIS2_PLACEMENT_3D('',#44327,#33829,#33830);
#29543=AXIS2_PLACEMENT_3D('',#44411,#33831,#33832);
#29544=AXIS2_PLACEMENT_3D('',#44429,#33834,#33835);
#29545=AXIS2_PLACEMENT_3D('',#44439,#33836,#33837);
#29546=AXIS2_PLACEMENT_3D('',#44477,#33839,#33840);
#29547=AXIS2_PLACEMENT_3D('',#44515,#33842,#33843);
#29548=AXIS2_PLACEMENT_3D('',#44553,#33845,#33846);
#29549=AXIS2_PLACEMENT_3D('',#44564,#33850,#33851);
#29550=AXIS2_PLACEMENT_3D('',#44572,#33854,#33855);
#29551=AXIS2_PLACEMENT_3D('',#44573,#33856,#33857);
#29552=AXIS2_PLACEMENT_3D('',#44574,#33858,#33859);
#29553=AXIS2_PLACEMENT_3D('',#44585,#33863,#33864);
#29554=AXIS2_PLACEMENT_3D('',#44593,#33867,#33868);
#29555=AXIS2_PLACEMENT_3D('',#44594,#33869,#33870);
#29556=AXIS2_PLACEMENT_3D('',#44595,#33871,#33872);
#29557=AXIS2_PLACEMENT_3D('',#44606,#33876,#33877);
#29558=AXIS2_PLACEMENT_3D('',#44614,#33880,#33881);
#29559=AXIS2_PLACEMENT_3D('',#44615,#33882,#33883);
#29560=AXIS2_PLACEMENT_3D('',#44616,#33884,#33885);
#29561=AXIS2_PLACEMENT_3D('',#44627,#33889,#33890);
#29562=AXIS2_PLACEMENT_3D('',#44635,#33893,#33894);
#29563=AXIS2_PLACEMENT_3D('',#44636,#33895,#33896);
#29564=AXIS2_PLACEMENT_3D('',#44637,#33897,#33898);
#29565=AXIS2_PLACEMENT_3D('',#44648,#33902,#33903);
#29566=AXIS2_PLACEMENT_3D('',#44656,#33906,#33907);
#29567=AXIS2_PLACEMENT_3D('',#44657,#33908,#33909);
#29568=AXIS2_PLACEMENT_3D('',#44658,#33910,#33911);
#29569=AXIS2_PLACEMENT_3D('',#44669,#33915,#33916);
#29570=AXIS2_PLACEMENT_3D('',#44677,#33919,#33920);
#29571=AXIS2_PLACEMENT_3D('',#44679,#33921,#33922);
#29572=AXIS2_PLACEMENT_3D('',#44680,#33923,#33924);
#29573=AXIS2_PLACEMENT_3D('',#44681,#33925,#33926);
#29574=AXIS2_PLACEMENT_3D('',#44692,#33930,#33931);
#29575=AXIS2_PLACEMENT_3D('',#44700,#33934,#33935);
#29576=AXIS2_PLACEMENT_3D('',#44701,#33936,#33937);
#29577=AXIS2_PLACEMENT_3D('',#44702,#33938,#33939);
#29578=AXIS2_PLACEMENT_3D('',#44713,#33943,#33944);
#29579=AXIS2_PLACEMENT_3D('',#44721,#33947,#33948);
#29580=AXIS2_PLACEMENT_3D('',#44722,#33949,#33950);
#29581=AXIS2_PLACEMENT_3D('',#44723,#33951,#33952);
#29582=AXIS2_PLACEMENT_3D('',#44734,#33956,#33957);
#29583=AXIS2_PLACEMENT_3D('',#44742,#33960,#33961);
#29584=AXIS2_PLACEMENT_3D('',#44743,#33962,#33963);
#29585=AXIS2_PLACEMENT_3D('',#44744,#33964,#33965);
#29586=AXIS2_PLACEMENT_3D('',#44755,#33969,#33970);
#29587=AXIS2_PLACEMENT_3D('',#44763,#33973,#33974);
#29588=AXIS2_PLACEMENT_3D('',#44764,#33975,#33976);
#29589=AXIS2_PLACEMENT_3D('',#44765,#33977,#33978);
#29590=AXIS2_PLACEMENT_3D('',#44776,#33982,#33983);
#29591=AXIS2_PLACEMENT_3D('',#44784,#33986,#33987);
#29592=AXIS2_PLACEMENT_3D('',#44785,#33988,#33989);
#29593=AXIS2_PLACEMENT_3D('',#44786,#33990,#33991);
#29594=AXIS2_PLACEMENT_3D('',#44797,#33995,#33996);
#29595=AXIS2_PLACEMENT_3D('',#44805,#33999,#34000);
#29596=AXIS2_PLACEMENT_3D('',#44806,#34001,#34002);
#29597=AXIS2_PLACEMENT_3D('',#44807,#34003,#34004);
#29598=AXIS2_PLACEMENT_3D('',#44818,#34008,#34009);
#29599=AXIS2_PLACEMENT_3D('',#44826,#34012,#34013);
#29600=AXIS2_PLACEMENT_3D('',#44827,#34014,#34015);
#29601=AXIS2_PLACEMENT_3D('',#44828,#34016,#34017);
#29602=AXIS2_PLACEMENT_3D('',#44839,#34021,#34022);
#29603=AXIS2_PLACEMENT_3D('',#44847,#34025,#34026);
#29604=AXIS2_PLACEMENT_3D('',#44848,#34027,#34028);
#29605=AXIS2_PLACEMENT_3D('',#44849,#34029,#34030);
#29606=AXIS2_PLACEMENT_3D('',#44860,#34034,#34035);
#29607=AXIS2_PLACEMENT_3D('',#44868,#34038,#34039);
#29608=AXIS2_PLACEMENT_3D('',#44869,#34040,#34041);
#29609=AXIS2_PLACEMENT_3D('',#44870,#34042,#34043);
#29610=AXIS2_PLACEMENT_3D('',#44881,#34047,#34048);
#29611=AXIS2_PLACEMENT_3D('',#44889,#34051,#34052);
#29612=AXIS2_PLACEMENT_3D('',#44890,#34053,#34054);
#29613=AXIS2_PLACEMENT_3D('',#44891,#34055,#34056);
#29614=AXIS2_PLACEMENT_3D('',#44902,#34060,#34061);
#29615=AXIS2_PLACEMENT_3D('',#44910,#34064,#34065);
#29616=AXIS2_PLACEMENT_3D('',#44911,#34066,#34067);
#29617=AXIS2_PLACEMENT_3D('',#44912,#34068,#34069);
#29618=AXIS2_PLACEMENT_3D('',#44923,#34073,#34074);
#29619=AXIS2_PLACEMENT_3D('',#44931,#34077,#34078);
#29620=AXIS2_PLACEMENT_3D('',#44932,#34079,#34080);
#29621=AXIS2_PLACEMENT_3D('',#44933,#34081,#34082);
#29622=AXIS2_PLACEMENT_3D('',#44944,#34086,#34087);
#29623=AXIS2_PLACEMENT_3D('',#44952,#34090,#34091);
#29624=AXIS2_PLACEMENT_3D('',#44953,#34092,#34093);
#29625=AXIS2_PLACEMENT_3D('',#44954,#34094,#34095);
#29626=AXIS2_PLACEMENT_3D('',#44965,#34099,#34100);
#29627=AXIS2_PLACEMENT_3D('',#44973,#34103,#34104);
#29628=AXIS2_PLACEMENT_3D('',#44974,#34105,#34106);
#29629=AXIS2_PLACEMENT_3D('',#44975,#34107,#34108);
#29630=AXIS2_PLACEMENT_3D('',#44986,#34112,#34113);
#29631=AXIS2_PLACEMENT_3D('',#44994,#34116,#34117);
#29632=AXIS2_PLACEMENT_3D('',#44995,#34118,#34119);
#29633=AXIS2_PLACEMENT_3D('',#44996,#34120,#34121);
#29634=AXIS2_PLACEMENT_3D('',#45007,#34125,#34126);
#29635=AXIS2_PLACEMENT_3D('',#45015,#34129,#34130);
#29636=AXIS2_PLACEMENT_3D('',#45016,#34131,#34132);
#29637=AXIS2_PLACEMENT_3D('',#45017,#34133,#34134);
#29638=AXIS2_PLACEMENT_3D('',#45028,#34138,#34139);
#29639=AXIS2_PLACEMENT_3D('',#45036,#34142,#34143);
#29640=AXIS2_PLACEMENT_3D('',#45037,#34144,#34145);
#29641=AXIS2_PLACEMENT_3D('',#45038,#34146,#34147);
#29642=AXIS2_PLACEMENT_3D('',#45049,#34151,#34152);
#29643=AXIS2_PLACEMENT_3D('',#45057,#34155,#34156);
#29644=AXIS2_PLACEMENT_3D('',#45058,#34157,#34158);
#29645=AXIS2_PLACEMENT_3D('',#45059,#34159,#34160);
#29646=AXIS2_PLACEMENT_3D('',#45061,#34161,#34162);
#29647=AXIS2_PLACEMENT_3D('',#45063,#34164,#34165);
#29648=AXIS2_PLACEMENT_3D('',#45064,#34166,#34167);
#29649=AXIS2_PLACEMENT_3D('',#45065,#34168,#34169);
#29650=AXIS2_PLACEMENT_3D('',#45066,#34170,#34171);
#29651=AXIS2_PLACEMENT_3D('',#45067,#34172,#34173);
#29652=AXIS2_PLACEMENT_3D('',#45068,#34174,#34175);
#29653=AXIS2_PLACEMENT_3D('',#45069,#34176,#34177);
#29654=AXIS2_PLACEMENT_3D('',#45070,#34178,#34179);
#29655=AXIS2_PLACEMENT_3D('',#45071,#34180,#34181);
#29656=AXIS2_PLACEMENT_3D('',#45072,#34182,#34183);
#29657=AXIS2_PLACEMENT_3D('',#45073,#34184,#34185);
#29658=AXIS2_PLACEMENT_3D('',#45074,#34186,#34187);
#29659=AXIS2_PLACEMENT_3D('',#45075,#34188,#34189);
#29660=AXIS2_PLACEMENT_3D('',#45076,#34190,#34191);
#29661=AXIS2_PLACEMENT_3D('',#45077,#34192,#34193);
#29662=AXIS2_PLACEMENT_3D('',#45078,#34194,#34195);
#29663=AXIS2_PLACEMENT_3D('',#45079,#34196,#34197);
#29664=AXIS2_PLACEMENT_3D('',#45080,#34198,#34199);
#29665=AXIS2_PLACEMENT_3D('',#45081,#34200,#34201);
#29666=AXIS2_PLACEMENT_3D('',#45082,#34202,#34203);
#29667=AXIS2_PLACEMENT_3D('',#45083,#34204,#34205);
#29668=AXIS2_PLACEMENT_3D('',#45084,#34206,#34207);
#29669=AXIS2_PLACEMENT_3D('',#45085,#34208,#34209);
#29670=AXIS2_PLACEMENT_3D('',#45086,#34210,#34211);
#29671=AXIS2_PLACEMENT_3D('',#45087,#34212,#34213);
#29672=AXIS2_PLACEMENT_3D('',#45088,#34214,#34215);
#29673=AXIS2_PLACEMENT_3D('',#45089,#34216,#34217);
#29674=AXIS2_PLACEMENT_3D('',#45090,#34218,#34219);
#29675=AXIS2_PLACEMENT_3D('',#45091,#34220,#34221);
#29676=AXIS2_PLACEMENT_3D('',#45092,#34222,#34223);
#29677=AXIS2_PLACEMENT_3D('',#45093,#34224,#34225);
#29678=AXIS2_PLACEMENT_3D('',#45094,#34226,#34227);
#29679=AXIS2_PLACEMENT_3D('',#45095,#34228,#34229);
#29680=AXIS2_PLACEMENT_3D('',#45096,#34230,#34231);
#29681=AXIS2_PLACEMENT_3D('',#45097,#34232,#34233);
#29682=AXIS2_PLACEMENT_3D('',#45098,#34234,#34235);
#29683=AXIS2_PLACEMENT_3D('',#45099,#34236,#34237);
#29684=AXIS2_PLACEMENT_3D('',#45100,#34238,#34239);
#29685=AXIS2_PLACEMENT_3D('',#45101,#34240,#34241);
#29686=AXIS2_PLACEMENT_3D('',#45102,#34242,#34243);
#29687=AXIS2_PLACEMENT_3D('',#45103,#34244,#34245);
#29688=AXIS2_PLACEMENT_3D('',#45104,#34246,#34247);
#29689=AXIS2_PLACEMENT_3D('',#45105,#34248,#34249);
#29690=AXIS2_PLACEMENT_3D('',#45106,#34250,#34251);
#29691=AXIS2_PLACEMENT_3D('',#45107,#34252,#34253);
#29692=AXIS2_PLACEMENT_3D('',#45108,#34254,#34255);
#29693=AXIS2_PLACEMENT_3D('',#45109,#34256,#34257);
#29694=AXIS2_PLACEMENT_3D('',#45110,#34258,#34259);
#29695=AXIS2_PLACEMENT_3D('',#45111,#34260,#34261);
#29696=AXIS2_PLACEMENT_3D('',#45112,#34262,#34263);
#29697=AXIS2_PLACEMENT_3D('',#45113,#34264,#34265);
#29698=AXIS2_PLACEMENT_3D('',#45114,#34266,#34267);
#29699=AXIS2_PLACEMENT_3D('',#45115,#34268,#34269);
#29700=AXIS2_PLACEMENT_3D('',#45116,#34270,#34271);
#29701=AXIS2_PLACEMENT_3D('',#45117,#34272,#34273);
#29702=AXIS2_PLACEMENT_3D('',#45118,#34274,#34275);
#29703=AXIS2_PLACEMENT_3D('',#45119,#34276,#34277);
#29704=AXIS2_PLACEMENT_3D('',#45120,#34278,#34279);
#29705=AXIS2_PLACEMENT_3D('',#45121,#34280,#34281);
#29706=AXIS2_PLACEMENT_3D('',#45122,#34282,#34283);
#29707=AXIS2_PLACEMENT_3D('',#45123,#34284,#34285);
#29708=AXIS2_PLACEMENT_3D('',#45124,#34286,#34287);
#29709=AXIS2_PLACEMENT_3D('',#45125,#34288,#34289);
#29710=AXIS2_PLACEMENT_3D('',#45126,#34290,#34291);
#29711=AXIS2_PLACEMENT_3D('',#45127,#34292,#34293);
#29712=AXIS2_PLACEMENT_3D('',#45128,#34294,#34295);
#29713=AXIS2_PLACEMENT_3D('',#45129,#34296,#34297);
#29714=AXIS2_PLACEMENT_3D('',#45130,#34298,#34299);
#29715=AXIS2_PLACEMENT_3D('',#45131,#34300,#34301);
#29716=AXIS2_PLACEMENT_3D('',#45132,#34302,#34303);
#29717=AXIS2_PLACEMENT_3D('',#45591,#34304,#34305);
#29718=AXIS2_PLACEMENT_3D('',#45593,#34306,#34307);
#29719=AXIS2_PLACEMENT_3D('',#46040,#34308,#34309);
#29720=AXIS2_PLACEMENT_3D('',#46041,#34310,#34311);
#29721=AXIS2_PLACEMENT_3D('',#46042,#34312,#34313);
#29722=AXIS2_PLACEMENT_3D('',#46044,#34314,#34315);
#29723=AXIS2_PLACEMENT_3D('',#46045,#34316,#34317);
#29724=AXIS2_PLACEMENT_3D('',#46047,#34318,#34319);
#29725=AXIS2_PLACEMENT_3D('',#46049,#34321,#34322);
#29726=AXIS2_PLACEMENT_3D('',#46051,#34323,#34324);
#29727=AXIS2_PLACEMENT_3D('',#46053,#34326,#34327);
#29728=AXIS2_PLACEMENT_3D('',#46055,#34328,#34329);
#29729=AXIS2_PLACEMENT_3D('',#46057,#34331,#34332);
#29730=AXIS2_PLACEMENT_3D('',#46058,#34333,#34334);
#29731=AXIS2_PLACEMENT_3D('',#46060,#34335,#34336);
#29732=AXIS2_PLACEMENT_3D('',#46061,#34337,#34338);
#29733=AXIS2_PLACEMENT_3D('',#46062,#34339,#34340);
#29734=AXIS2_PLACEMENT_3D('',#46064,#34342,#34343);
#29735=AXIS2_PLACEMENT_3D('',#46065,#34344,#34345);
#33810=DIRECTION('axis',(0.,0.,1.));
#33811=DIRECTION('refdir',(1.,0.,0.));
#33812=DIRECTION('center_axis',(0.,0.,1.));
#33813=DIRECTION('ref_axis',(-0.532340283278114,0.846530461826022,0.));
#33814=DIRECTION('',(0.,0.,-1.));
#33815=DIRECTION('center_axis',(0.,0.,-1.));
#33816=DIRECTION('ref_axis',(1.,0.,0.));
#33817=DIRECTION('center_axis',(0.,0.,1.));
#33818=DIRECTION('ref_axis',(1.,0.,0.));
#33819=DIRECTION('',(0.,0.,-1.));
#33820=DIRECTION('center_axis',(0.,0.,1.));
#33821=DIRECTION('ref_axis',(1.,0.,0.));
#33822=DIRECTION('',(0.,0.,-1.));
#33823=DIRECTION('center_axis',(0.,0.,1.));
#33824=DIRECTION('ref_axis',(1.,0.,0.));
#33825=DIRECTION('',(0.,0.,-1.));
#33826=DIRECTION('center_axis',(0.,0.,1.));
#33827=DIRECTION('ref_axis',(1.,0.,0.));
#33828=DIRECTION('',(0.,0.,-1.));
#33829=DIRECTION('center_axis',(0.,0.,1.));
#33830=DIRECTION('ref_axis',(1.,0.,0.));
#33831=DIRECTION('center_axis',(0.,0.,1.));
#33832=DIRECTION('ref_axis',(0.409460327591604,-0.91232792357166,0.));
#33833=DIRECTION('',(0.,0.,1.));
#33834=DIRECTION('center_axis',(0.,0.,1.));
#33835=DIRECTION('ref_axis',(1.,-5.87495706799284E-15,0.));
#33836=DIRECTION('center_axis',(0.,0.,1.));
#33837=DIRECTION('ref_axis',(1.,-5.87495706799284E-15,0.));
#33838=DIRECTION('',(0.,0.,1.));
#33839=DIRECTION('center_axis',(0.,0.,1.));
#33840=DIRECTION('ref_axis',(1.,-5.87495706799284E-15,0.));
#33841=DIRECTION('',(0.,0.,1.));
#33842=DIRECTION('center_axis',(0.,0.,1.));
#33843=DIRECTION('ref_axis',(1.,-5.87495706799284E-15,0.));
#33844=DIRECTION('',(0.,0.,1.));
#33845=DIRECTION('center_axis',(-0.993575558391583,-0.113170710728767,0.));
#33846=DIRECTION('ref_axis',(-0.113170710728767,0.993575558391583,0.));
#33847=DIRECTION('',(0.,0.,1.));
#33848=DIRECTION('',(-0.113170710728767,0.993575558391583,0.));
#33849=DIRECTION('',(0.,0.,-1.));
#33850=DIRECTION('center_axis',(-0.398779068740344,0.917047029510801,0.));
#33851=DIRECTION('ref_axis',(0.917047029510801,0.398779068740344,0.));
#33852=DIRECTION('',(0.917047029510801,0.398779068740344,0.));
#33853=DIRECTION('',(0.,0.,-1.));
#33854=DIRECTION('center_axis',(0.,0.,-1.));
#33855=DIRECTION('ref_axis',(-1.,0.,0.));
#33856=DIRECTION('center_axis',(0.,0.,1.));
#33857=DIRECTION('ref_axis',(1.,0.,0.));
#33858=DIRECTION('center_axis',(-0.917047029510801,0.398779068740345,0.));
#33859=DIRECTION('ref_axis',(0.398779068740345,0.917047029510801,0.));
#33860=DIRECTION('',(0.,0.,1.));
#33861=DIRECTION('',(0.398779068740345,0.917047029510801,0.));
#33862=DIRECTION('',(0.,0.,-1.));
#33863=DIRECTION('center_axis',(0.113170710728767,0.993575558391583,0.));
#33864=DIRECTION('ref_axis',(0.993575558391583,-0.113170710728767,0.));
#33865=DIRECTION('',(0.993575558391583,-0.113170710728767,0.));
#33866=DIRECTION('',(0.,0.,-1.));
#33867=DIRECTION('center_axis',(0.,0.,-1.));
#33868=DIRECTION('ref_axis',(-1.,0.,0.));
#33869=DIRECTION('center_axis',(0.,0.,1.));
#33870=DIRECTION('ref_axis',(1.,0.,0.));
#33871=DIRECTION('center_axis',(-0.594796489651244,0.803876318782036,0.));
#33872=DIRECTION('ref_axis',(0.803876318782036,0.594796489651244,0.));
#33873=DIRECTION('',(0.,0.,1.));
#33874=DIRECTION('',(0.803876318782036,0.594796489651244,0.));
#33875=DIRECTION('',(0.,0.,-1.));
#33876=DIRECTION('center_axis',(0.594796489651239,0.803876318782039,0.));
#33877=DIRECTION('ref_axis',(0.803876318782039,-0.594796489651239,0.));
#33878=DIRECTION('',(0.803876318782039,-0.594796489651239,0.));
#33879=DIRECTION('',(0.,0.,-1.));
#33880=DIRECTION('center_axis',(0.,0.,-1.));
#33881=DIRECTION('ref_axis',(-1.,0.,0.));
#33882=DIRECTION('center_axis',(0.,0.,1.));
#33883=DIRECTION('ref_axis',(1.,0.,0.));
#33884=DIRECTION('center_axis',(-0.113170710728767,0.993575558391583,0.));
#33885=DIRECTION('ref_axis',(0.993575558391583,0.113170710728767,0.));
#33886=DIRECTION('',(0.,0.,1.));
#33887=DIRECTION('',(0.993575558391583,0.113170710728767,0.));
#33888=DIRECTION('',(0.,0.,-1.));
#33889=DIRECTION('center_axis',(0.917047029510801,0.398779068740344,0.));
#33890=DIRECTION('ref_axis',(0.398779068740344,-0.917047029510801,0.));
#33891=DIRECTION('',(0.398779068740344,-0.917047029510801,0.));
#33892=DIRECTION('',(0.,0.,-1.));
#33893=DIRECTION('center_axis',(0.,0.,-1.));
#33894=DIRECTION('ref_axis',(-1.,0.,0.));
#33895=DIRECTION('center_axis',(0.,0.,1.));
#33896=DIRECTION('ref_axis',(1.,0.,0.));
#33897=DIRECTION('center_axis',(0.398779068740341,0.917047029510803,0.));
#33898=DIRECTION('ref_axis',(0.917047029510803,-0.398779068740341,0.));
#33899=DIRECTION('',(0.,0.,1.));
#33900=DIRECTION('',(0.917047029510803,-0.398779068740341,0.));
#33901=DIRECTION('',(0.,0.,-1.));
#33902=DIRECTION('center_axis',(0.993575558391583,-0.113170710728765,0.));
#33903=DIRECTION('ref_axis',(-0.113170710728765,-0.993575558391583,0.));
#33904=DIRECTION('',(-0.113170710728765,-0.993575558391583,0.));
#33905=DIRECTION('',(0.,0.,-1.));
#33906=DIRECTION('center_axis',(0.,0.,-1.));
#33907=DIRECTION('ref_axis',(-1.,0.,0.));
#33908=DIRECTION('center_axis',(0.,0.,1.));
#33909=DIRECTION('ref_axis',(1.,0.,0.));
#33910=DIRECTION('center_axis',(0.803876318782038,0.594796489651242,0.));
#33911=DIRECTION('ref_axis',(0.594796489651242,-0.803876318782038,0.));
#33912=DIRECTION('',(0.,0.,1.));
#33913=DIRECTION('',(0.594796489651242,-0.803876318782038,0.));
#33914=DIRECTION('',(0.,0.,-1.));
#33915=DIRECTION('center_axis',(0.803876318782038,-0.594796489651242,0.));
#33916=DIRECTION('ref_axis',(-0.594796489651242,-0.803876318782038,0.));
#33917=DIRECTION('',(-0.594796489651242,-0.803876318782038,0.));
#33918=DIRECTION('',(0.,0.,-1.));
#33919=DIRECTION('center_axis',(0.,0.,-1.));
#33920=DIRECTION('ref_axis',(-1.,0.,0.));
#33921=DIRECTION('center_axis',(0.,0.,1.));
#33922=DIRECTION('ref_axis',(1.,0.,0.));
#33923=DIRECTION('center_axis',(0.,0.,1.));
#33924=DIRECTION('ref_axis',(1.,0.,0.));
#33925=DIRECTION('center_axis',(0.930429556935621,0.366470789532515,0.));
#33926=DIRECTION('ref_axis',(0.366470789532515,-0.930429556935621,0.));
#33927=DIRECTION('',(0.,0.,1.));
#33928=DIRECTION('',(0.366470789532515,-0.930429556935621,0.));
#33929=DIRECTION('',(0.,0.,-1.));
#33930=DIRECTION('center_axis',(0.622540237971889,-0.782587791947909,0.));
#33931=DIRECTION('ref_axis',(-0.782587791947909,-0.622540237971889,0.));
#33932=DIRECTION('',(-0.782587791947909,-0.622540237971889,0.));
#33933=DIRECTION('',(0.,0.,-1.));
#33934=DIRECTION('center_axis',(0.,0.,-1.));
#33935=DIRECTION('ref_axis',(-1.,0.,0.));
#33936=DIRECTION('center_axis',(0.,0.,1.));
#33937=DIRECTION('ref_axis',(1.,0.,0.));
#33938=DIRECTION('center_axis',(0.989011027504405,-0.147841764987712,0.));
#33939=DIRECTION('ref_axis',(-0.147841764987712,-0.989011027504405,0.));
#33940=DIRECTION('',(0.,0.,1.));
#33941=DIRECTION('',(-0.147841764987712,-0.989011027504405,0.));
#33942=DIRECTION('',(0.,0.,-1.));
#33943=DIRECTION('center_axis',(0.14784176498771,-0.989011027504405,0.));
#33944=DIRECTION('ref_axis',(-0.989011027504405,-0.14784176498771,0.));
#33945=DIRECTION('',(-0.989011027504405,-0.14784176498771,0.));
#33946=DIRECTION('',(0.,0.,-1.));
#33947=DIRECTION('center_axis',(0.,0.,-1.));
#33948=DIRECTION('ref_axis',(-1.,0.,0.));
#33949=DIRECTION('center_axis',(0.,0.,1.));
#33950=DIRECTION('ref_axis',(1.,0.,0.));
#33951=DIRECTION('center_axis',(0.782587791947909,-0.622540237971889,0.));
#33952=DIRECTION('ref_axis',(-0.622540237971889,-0.782587791947909,0.));
#33953=DIRECTION('',(0.,0.,1.));
#33954=DIRECTION('',(-0.622540237971889,-0.782587791947909,0.));
#33955=DIRECTION('',(0.,0.,-1.));
#33956=DIRECTION('center_axis',(-0.366470789532515,-0.930429556935621,0.));
#33957=DIRECTION('ref_axis',(-0.930429556935621,0.366470789532515,0.));
#33958=DIRECTION('',(-0.930429556935621,0.366470789532515,0.));
#33959=DIRECTION('',(0.,0.,-1.));
#33960=DIRECTION('center_axis',(0.,0.,-1.));
#33961=DIRECTION('ref_axis',(-1.,0.,0.));
#33962=DIRECTION('center_axis',(0.,0.,1.));
#33963=DIRECTION('ref_axis',(1.,0.,0.));
#33964=DIRECTION('center_axis',(0.366470789532517,-0.93042955693562,0.));
#33965=DIRECTION('ref_axis',(-0.93042955693562,-0.366470789532517,0.));
#33966=DIRECTION('',(0.,0.,1.));
#33967=DIRECTION('',(-0.93042955693562,-0.366470789532517,0.));
#33968=DIRECTION('',(0.,0.,-1.));
#33969=DIRECTION('center_axis',(-0.782587791947909,-0.622540237971889,0.));
#33970=DIRECTION('ref_axis',(-0.622540237971889,0.782587791947909,0.));
#33971=DIRECTION('',(-0.622540237971889,0.782587791947909,0.));
#33972=DIRECTION('',(0.,0.,-1.));
#33973=DIRECTION('center_axis',(0.,0.,-1.));
#33974=DIRECTION('ref_axis',(-1.,0.,0.));
#33975=DIRECTION('center_axis',(0.,0.,1.));
#33976=DIRECTION('ref_axis',(1.,0.,0.));
#33977=DIRECTION('center_axis',(-0.147841764987711,-0.989011027504405,0.));
#33978=DIRECTION('ref_axis',(-0.989011027504405,0.147841764987711,0.));
#33979=DIRECTION('',(0.,0.,1.));
#33980=DIRECTION('',(-0.989011027504405,0.147841764987711,0.));
#33981=DIRECTION('',(0.,0.,-1.));
#33982=DIRECTION('center_axis',(-0.989011027504405,-0.147841764987711,0.));
#33983=DIRECTION('ref_axis',(-0.147841764987711,0.989011027504405,0.));
#33984=DIRECTION('',(-0.147841764987711,0.989011027504405,0.));
#33985=DIRECTION('',(0.,0.,-1.));
#33986=DIRECTION('center_axis',(0.,0.,-1.));
#33987=DIRECTION('ref_axis',(-1.,0.,0.));
#33988=DIRECTION('center_axis',(0.,0.,1.));
#33989=DIRECTION('ref_axis',(1.,0.,0.));
#33990=DIRECTION('center_axis',(-0.622540237971888,-0.78258779194791,0.));
#33991=DIRECTION('ref_axis',(-0.78258779194791,0.622540237971888,0.));
#33992=DIRECTION('',(0.,0.,1.));
#33993=DIRECTION('',(-0.78258779194791,0.622540237971888,0.));
#33994=DIRECTION('',(0.,0.,-1.));
#33995=DIRECTION('center_axis',(-0.93042955693562,0.366470789532517,0.));
#33996=DIRECTION('ref_axis',(0.366470789532517,0.93042955693562,0.));
#33997=DIRECTION('',(0.366470789532517,0.93042955693562,0.));
#33998=DIRECTION('',(0.,0.,-1.));
#33999=DIRECTION('center_axis',(0.,0.,-1.));
#34000=DIRECTION('ref_axis',(-1.,0.,0.));
#34001=DIRECTION('center_axis',(0.,0.,1.));
#34002=DIRECTION('ref_axis',(1.,0.,0.));
#34003=DIRECTION('center_axis',(-0.398779068740341,-0.917047029510803,0.));
#34004=DIRECTION('ref_axis',(-0.917047029510803,0.398779068740341,0.));
#34005=DIRECTION('',(0.,0.,1.));
#34006=DIRECTION('',(-0.917047029510803,0.398779068740341,0.));
#34007=DIRECTION('',(0.,0.,-1.));
#34008=DIRECTION('center_axis',(-0.993575558391583,0.113170710728763,0.));
#34009=DIRECTION('ref_axis',(0.113170710728763,0.993575558391583,0.));
#34010=DIRECTION('',(0.113170710728763,0.993575558391583,0.));
#34011=DIRECTION('',(0.,0.,-1.));
#34012=DIRECTION('center_axis',(0.,0.,-1.));
#34013=DIRECTION('ref_axis',(-1.,0.,0.));
#34014=DIRECTION('center_axis',(0.,0.,1.));
#34015=DIRECTION('ref_axis',(1.,0.,0.));
#34016=DIRECTION('center_axis',(0.113170710728765,-0.993575558391583,0.));
#34017=DIRECTION('ref_axis',(-0.993575558391583,-0.113170710728765,0.));
#34018=DIRECTION('',(0.,0.,1.));
#34019=DIRECTION('',(-0.993575558391583,-0.113170710728765,0.));
#34020=DIRECTION('',(0.,0.,-1.));
#34021=DIRECTION('center_axis',(-0.917047029510802,-0.398779068740342,0.));
#34022=DIRECTION('ref_axis',(-0.398779068740342,0.917047029510802,0.));
#34023=DIRECTION('',(-0.398779068740342,0.917047029510802,0.));
#34024=DIRECTION('',(0.,0.,-1.));
#34025=DIRECTION('center_axis',(0.,0.,-1.));
#34026=DIRECTION('ref_axis',(-1.,0.,0.));
#34027=DIRECTION('center_axis',(0.,0.,1.));
#34028=DIRECTION('ref_axis',(1.,0.,0.));
#34029=DIRECTION('center_axis',(0.594796489651242,-0.803876318782038,0.));
#34030=DIRECTION('ref_axis',(-0.803876318782038,-0.594796489651242,0.));
#34031=DIRECTION('',(0.,0.,1.));
#34032=DIRECTION('',(-0.803876318782038,-0.594796489651242,0.));
#34033=DIRECTION('',(0.,0.,-1.));
#34034=DIRECTION('center_axis',(-0.594796489651242,-0.803876318782038,0.));
#34035=DIRECTION('ref_axis',(-0.803876318782038,0.594796489651242,0.));
#34036=DIRECTION('',(-0.803876318782038,0.594796489651242,0.));
#34037=DIRECTION('',(0.,0.,-1.));
#34038=DIRECTION('center_axis',(0.,0.,-1.));
#34039=DIRECTION('ref_axis',(-1.,0.,0.));
#34040=DIRECTION('center_axis',(0.,0.,1.));
#34041=DIRECTION('ref_axis',(1.,0.,0.));
#34042=DIRECTION('center_axis',(0.917047029510802,-0.398779068740341,0.));
#34043=DIRECTION('ref_axis',(-0.398779068740341,-0.917047029510802,0.));
#34044=DIRECTION('',(0.,0.,1.));
#34045=DIRECTION('',(-0.398779068740341,-0.917047029510802,0.));
#34046=DIRECTION('',(0.,0.,-1.));
#34047=DIRECTION('center_axis',(-0.113170710728766,-0.993575558391583,0.));
#34048=DIRECTION('ref_axis',(-0.993575558391583,0.113170710728766,0.));
#34049=DIRECTION('',(-0.993575558391583,0.113170710728766,0.));
#34050=DIRECTION('',(0.,0.,-1.));
#34051=DIRECTION('center_axis',(0.,0.,-1.));
#34052=DIRECTION('ref_axis',(-1.,0.,0.));
#34053=DIRECTION('center_axis',(0.,0.,1.));
#34054=DIRECTION('ref_axis',(1.,0.,0.));
#34055=DIRECTION('center_axis',(0.993575558391583,0.113170710728763,0.));
#34056=DIRECTION('ref_axis',(0.113170710728763,-0.993575558391583,0.));
#34057=DIRECTION('',(0.,0.,1.));
#34058=DIRECTION('',(0.113170710728763,-0.993575558391583,0.));
#34059=DIRECTION('',(0.,0.,-1.));
#34060=DIRECTION('center_axis',(0.398779068740342,-0.917047029510802,0.));
#34061=DIRECTION('ref_axis',(-0.917047029510802,-0.398779068740342,0.));
#34062=DIRECTION('',(-0.917047029510802,-0.398779068740342,0.));
#34063=DIRECTION('',(0.,0.,-1.));
#34064=DIRECTION('center_axis',(0.,0.,-1.));
#34065=DIRECTION('ref_axis',(-1.,0.,0.));
#34066=DIRECTION('center_axis',(0.,0.,1.));
#34067=DIRECTION('ref_axis',(1.,0.,0.));
#34068=DIRECTION('center_axis',(-0.803876318782038,-0.594796489651242,0.));
#34069=DIRECTION('ref_axis',(-0.594796489651242,0.803876318782038,0.));
#34070=DIRECTION('',(0.,0.,1.));
#34071=DIRECTION('',(-0.594796489651242,0.803876318782038,0.));
#34072=DIRECTION('',(0.,0.,-1.));
#34073=DIRECTION('center_axis',(-0.803876318782038,0.594796489651242,0.));
#34074=DIRECTION('ref_axis',(0.594796489651242,0.803876318782038,0.));
#34075=DIRECTION('',(0.594796489651242,0.803876318782038,0.));
#34076=DIRECTION('',(0.,0.,-1.));
#34077=DIRECTION('center_axis',(0.,0.,-1.));
#34078=DIRECTION('ref_axis',(-1.,0.,0.));
#34079=DIRECTION('center_axis',(0.,0.,1.));
#34080=DIRECTION('ref_axis',(1.,0.,0.));
#34081=DIRECTION('center_axis',(0.622540237971889,0.782587791947909,0.));
#34082=DIRECTION('ref_axis',(0.782587791947909,-0.622540237971889,0.));
#34083=DIRECTION('',(0.,0.,1.));
#34084=DIRECTION('',(0.782587791947909,-0.622540237971889,0.));
#34085=DIRECTION('',(0.,0.,-1.));
#34086=DIRECTION('center_axis',(0.93042955693562,-0.366470789532517,0.));
#34087=DIRECTION('ref_axis',(-0.366470789532517,-0.93042955693562,0.));
#34088=DIRECTION('',(-0.366470789532517,-0.93042955693562,0.));
#34089=DIRECTION('',(0.,0.,-1.));
#34090=DIRECTION('center_axis',(0.,0.,-1.));
#34091=DIRECTION('ref_axis',(-1.,0.,0.));
#34092=DIRECTION('center_axis',(0.,0.,1.));
#34093=DIRECTION('ref_axis',(1.,0.,0.));
#34094=DIRECTION('center_axis',(0.147841764987712,0.989011027504405,0.));
#34095=DIRECTION('ref_axis',(0.989011027504405,-0.147841764987712,0.));
#34096=DIRECTION('',(0.,0.,1.));
#34097=DIRECTION('',(0.989011027504405,-0.147841764987712,0.));
#34098=DIRECTION('',(0.,0.,-1.));
#34099=DIRECTION('center_axis',(0.989011027504404,0.147841764987713,0.));
#34100=DIRECTION('ref_axis',(0.147841764987713,-0.989011027504404,0.));
#34101=DIRECTION('',(0.147841764987713,-0.989011027504404,0.));
#34102=DIRECTION('',(0.,0.,-1.));
#34103=DIRECTION('center_axis',(0.,0.,-1.));
#34104=DIRECTION('ref_axis',(-1.,0.,0.));
#34105=DIRECTION('center_axis',(0.,0.,1.));
#34106=DIRECTION('ref_axis',(1.,0.,0.));
#34107=DIRECTION('center_axis',(-0.366470789532514,0.930429556935621,0.));
#34108=DIRECTION('ref_axis',(0.930429556935621,0.366470789532514,0.));
#34109=DIRECTION('',(0.,0.,1.));
#34110=DIRECTION('',(0.930429556935621,0.366470789532514,0.));
#34111=DIRECTION('',(0.,0.,-1.));
#34112=DIRECTION('center_axis',(0.782587791947912,0.622540237971886,0.));
#34113=DIRECTION('ref_axis',(0.622540237971886,-0.782587791947912,0.));
#34114=DIRECTION('',(0.622540237971886,-0.782587791947912,0.));
#34115=DIRECTION('',(0.,0.,-1.));
#34116=DIRECTION('center_axis',(0.,0.,-1.));
#34117=DIRECTION('ref_axis',(-1.,0.,0.));
#34118=DIRECTION('center_axis',(0.,0.,1.));
#34119=DIRECTION('ref_axis',(1.,0.,0.));
#34120=DIRECTION('center_axis',(-0.782587791947911,0.622540237971887,0.));
#34121=DIRECTION('ref_axis',(0.622540237971887,0.782587791947911,0.));
#34122=DIRECTION('',(0.,0.,1.));
#34123=DIRECTION('',(0.622540237971887,0.782587791947911,0.));
#34124=DIRECTION('',(0.,0.,-1.));
#34125=DIRECTION('center_axis',(0.366470789532514,0.930429556935621,0.));
#34126=DIRECTION('ref_axis',(0.930429556935621,-0.366470789532514,0.));
#34127=DIRECTION('',(0.930429556935621,-0.366470789532514,0.));
#34128=DIRECTION('',(0.,0.,-1.));
#34129=DIRECTION('center_axis',(0.,0.,-1.));
#34130=DIRECTION('ref_axis',(-1.,0.,0.));
#34131=DIRECTION('center_axis',(0.,0.,1.));
#34132=DIRECTION('ref_axis',(1.,0.,0.));
#34133=DIRECTION('center_axis',(-0.989011027504405,0.147841764987707,0.));
#34134=DIRECTION('ref_axis',(0.147841764987707,0.989011027504405,0.));
#34135=DIRECTION('',(0.,0.,1.));
#34136=DIRECTION('',(0.147841764987707,0.989011027504405,0.));
#34137=DIRECTION('',(0.,0.,-1.));
#34138=DIRECTION('center_axis',(-0.147841764987713,0.989011027504404,0.));
#34139=DIRECTION('ref_axis',(0.989011027504404,0.147841764987713,0.));
#34140=DIRECTION('',(0.989011027504404,0.147841764987713,0.));
#34141=DIRECTION('',(0.,0.,-1.));
#34142=DIRECTION('center_axis',(0.,0.,-1.));
#34143=DIRECTION('ref_axis',(-1.,0.,0.));
#34144=DIRECTION('center_axis',(0.,0.,1.));
#34145=DIRECTION('ref_axis',(1.,0.,0.));
#34146=DIRECTION('center_axis',(-0.930429556935621,-0.366470789532514,0.));
#34147=DIRECTION('ref_axis',(-0.366470789532514,0.930429556935621,0.));
#34148=DIRECTION('',(0.,0.,1.));
#34149=DIRECTION('',(-0.366470789532514,0.930429556935621,0.));
#34150=DIRECTION('',(0.,0.,-1.));
#34151=DIRECTION('center_axis',(-0.622540237971886,0.782587791947912,0.));
#34152=DIRECTION('ref_axis',(0.782587791947912,0.622540237971886,0.));
#34153=DIRECTION('',(0.782587791947912,0.622540237971886,0.));
#34154=DIRECTION('',(0.,0.,-1.));
#34155=DIRECTION('center_axis',(0.,0.,-1.));
#34156=DIRECTION('ref_axis',(-1.,0.,0.));
#34157=DIRECTION('center_axis',(0.,0.,1.));
#34158=DIRECTION('ref_axis',(1.,0.,0.));
#34159=DIRECTION('center_axis',(0.,0.,-1.));
#34160=DIRECTION('ref_axis',(1.,0.,0.));
#34161=DIRECTION('center_axis',(0.,0.,1.));
#34162=DIRECTION('ref_axis',(1.,0.,0.));
#34163=DIRECTION('',(-0.707106781186534,-8.65956056235477E-17,-0.707106781186561));
#34164=DIRECTION('center_axis',(0.,0.,1.));
#34165=DIRECTION('ref_axis',(1.,0.,0.));
#34166=DIRECTION('center_axis',(0.,0.,1.));
#34167=DIRECTION('ref_axis',(1.,0.,0.));
#34168=DIRECTION('center_axis',(0.,0.,1.));
#34169=DIRECTION('ref_axis',(1.,0.,0.));
#34170=DIRECTION('center_axis',(0.,0.,1.));
#34171=DIRECTION('ref_axis',(1.,0.,0.));
#34172=DIRECTION('center_axis',(0.,0.,1.));
#34173=DIRECTION('ref_axis',(1.,0.,0.));
#34174=DIRECTION('center_axis',(0.,0.,1.));
#34175=DIRECTION('ref_axis',(1.,0.,0.));
#34176=DIRECTION('center_axis',(0.,0.,1.));
#34177=DIRECTION('ref_axis',(1.,0.,0.));
#34178=DIRECTION('center_axis',(0.,0.,1.));
#34179=DIRECTION('ref_axis',(1.,0.,0.));
#34180=DIRECTION('center_axis',(0.,0.,1.));
#34181=DIRECTION('ref_axis',(1.,0.,0.));
#34182=DIRECTION('center_axis',(0.,0.,1.));
#34183=DIRECTION('ref_axis',(1.,0.,0.));
#34184=DIRECTION('center_axis',(0.,0.,1.));
#34185=DIRECTION('ref_axis',(1.,0.,0.));
#34186=DIRECTION('center_axis',(0.,0.,1.));
#34187=DIRECTION('ref_axis',(1.,0.,0.));
#34188=DIRECTION('center_axis',(0.,0.,1.));
#34189=DIRECTION('ref_axis',(1.,0.,0.));
#34190=DIRECTION('center_axis',(0.,0.,1.));
#34191=DIRECTION('ref_axis',(1.,0.,0.));
#34192=DIRECTION('center_axis',(0.,0.,1.));
#34193=DIRECTION('ref_axis',(1.,0.,0.));
#34194=DIRECTION('center_axis',(0.,0.,1.));
#34195=DIRECTION('ref_axis',(1.,0.,0.));
#34196=DIRECTION('center_axis',(0.,0.,1.));
#34197=DIRECTION('ref_axis',(1.,0.,0.));
#34198=DIRECTION('center_axis',(0.,0.,1.));
#34199=DIRECTION('ref_axis',(1.,0.,0.));
#34200=DIRECTION('center_axis',(0.,0.,1.));
#34201=DIRECTION('ref_axis',(1.,0.,0.));
#34202=DIRECTION('center_axis',(0.,0.,1.));
#34203=DIRECTION('ref_axis',(1.,0.,0.));
#34204=DIRECTION('center_axis',(0.,0.,1.));
#34205=DIRECTION('ref_axis',(1.,0.,0.));
#34206=DIRECTION('center_axis',(0.,0.,1.));
#34207=DIRECTION('ref_axis',(1.,0.,0.));
#34208=DIRECTION('center_axis',(0.,0.,1.));
#34209=DIRECTION('ref_axis',(1.,0.,0.));
#34210=DIRECTION('center_axis',(0.,0.,1.));
#34211=DIRECTION('ref_axis',(1.,0.,0.));
#34212=DIRECTION('center_axis',(0.,0.,1.));
#34213=DIRECTION('ref_axis',(1.,0.,0.));
#34214=DIRECTION('center_axis',(0.,0.,1.));
#34215=DIRECTION('ref_axis',(1.,0.,0.));
#34216=DIRECTION('center_axis',(0.,0.,1.));
#34217=DIRECTION('ref_axis',(1.,0.,0.));
#34218=DIRECTION('center_axis',(0.,0.,1.));
#34219=DIRECTION('ref_axis',(1.,0.,0.));
#34220=DIRECTION('center_axis',(0.,0.,1.));
#34221=DIRECTION('ref_axis',(1.,0.,0.));
#34222=DIRECTION('center_axis',(0.,0.,1.));
#34223=DIRECTION('ref_axis',(1.,0.,0.));
#34224=DIRECTION('center_axis',(0.,0.,1.));
#34225=DIRECTION('ref_axis',(1.,0.,0.));
#34226=DIRECTION('center_axis',(0.,0.,1.));
#34227=DIRECTION('ref_axis',(1.,0.,0.));
#34228=DIRECTION('center_axis',(0.,0.,1.));
#34229=DIRECTION('ref_axis',(1.,0.,0.));
#34230=DIRECTION('center_axis',(0.,0.,1.));
#34231=DIRECTION('ref_axis',(1.,0.,0.));
#34232=DIRECTION('center_axis',(0.,0.,1.));
#34233=DIRECTION('ref_axis',(1.,0.,0.));
#34234=DIRECTION('center_axis',(0.,0.,1.));
#34235=DIRECTION('ref_axis',(1.,0.,0.));
#34236=DIRECTION('center_axis',(0.,0.,1.));
#34237=DIRECTION('ref_axis',(1.,0.,0.));
#34238=DIRECTION('center_axis',(0.,0.,1.));
#34239=DIRECTION('ref_axis',(1.,0.,0.));
#34240=DIRECTION('center_axis',(0.,0.,1.));
#34241=DIRECTION('ref_axis',(1.,0.,0.));
#34242=DIRECTION('center_axis',(0.,0.,1.));
#34243=DIRECTION('ref_axis',(1.,0.,0.));
#34244=DIRECTION('center_axis',(0.,0.,1.));
#34245=DIRECTION('ref_axis',(1.,0.,0.));
#34246=DIRECTION('center_axis',(0.,0.,1.));
#34247=DIRECTION('ref_axis',(1.,0.,0.));
#34248=DIRECTION('center_axis',(0.,0.,1.));
#34249=DIRECTION('ref_axis',(1.,0.,0.));
#34250=DIRECTION('center_axis',(0.,0.,1.));
#34251=DIRECTION('ref_axis',(1.,0.,0.));
#34252=DIRECTION('center_axis',(0.,0.,1.));
#34253=DIRECTION('ref_axis',(1.,0.,0.));
#34254=DIRECTION('center_axis',(0.,0.,1.));
#34255=DIRECTION('ref_axis',(1.,0.,0.));
#34256=DIRECTION('center_axis',(0.,0.,1.));
#34257=DIRECTION('ref_axis',(1.,0.,0.));
#34258=DIRECTION('center_axis',(0.,0.,1.));
#34259=DIRECTION('ref_axis',(1.,0.,0.));
#34260=DIRECTION('center_axis',(0.,0.,1.));
#34261=DIRECTION('ref_axis',(1.,0.,0.));
#34262=DIRECTION('center_axis',(0.,0.,1.));
#34263=DIRECTION('ref_axis',(1.,0.,0.));
#34264=DIRECTION('center_axis',(0.,0.,1.));
#34265=DIRECTION('ref_axis',(1.,0.,0.));
#34266=DIRECTION('center_axis',(0.,0.,1.));
#34267=DIRECTION('ref_axis',(1.,0.,0.));
#34268=DIRECTION('center_axis',(0.,0.,1.));
#34269=DIRECTION('ref_axis',(1.,0.,0.));
#34270=DIRECTION('center_axis',(0.,0.,1.));
#34271=DIRECTION('ref_axis',(1.,0.,0.));
#34272=DIRECTION('center_axis',(0.,0.,1.));
#34273=DIRECTION('ref_axis',(1.,0.,0.));
#34274=DIRECTION('center_axis',(0.,0.,1.));
#34275=DIRECTION('ref_axis',(1.,0.,0.));
#34276=DIRECTION('center_axis',(0.,0.,1.));
#34277=DIRECTION('ref_axis',(1.,0.,0.));
#34278=DIRECTION('center_axis',(0.,0.,1.));
#34279=DIRECTION('ref_axis',(1.,0.,0.));
#34280=DIRECTION('center_axis',(0.,0.,1.));
#34281=DIRECTION('ref_axis',(1.,0.,0.));
#34282=DIRECTION('center_axis',(0.,0.,1.));
#34283=DIRECTION('ref_axis',(1.,0.,0.));
#34284=DIRECTION('center_axis',(0.,0.,1.));
#34285=DIRECTION('ref_axis',(1.,0.,0.));
#34286=DIRECTION('center_axis',(0.,0.,1.));
#34287=DIRECTION('ref_axis',(1.,0.,0.));
#34288=DIRECTION('center_axis',(0.,0.,1.));
#34289=DIRECTION('ref_axis',(1.,0.,0.));
#34290=DIRECTION('center_axis',(0.,0.,1.));
#34291=DIRECTION('ref_axis',(1.,0.,0.));
#34292=DIRECTION('center_axis',(0.,0.,1.));
#34293=DIRECTION('ref_axis',(1.,0.,0.));
#34294=DIRECTION('center_axis',(0.,0.,1.));
#34295=DIRECTION('ref_axis',(1.,0.,0.));
#34296=DIRECTION('center_axis',(0.,0.,1.));
#34297=DIRECTION('ref_axis',(1.,0.,0.));
#34298=DIRECTION('center_axis',(0.,0.,1.));
#34299=DIRECTION('ref_axis',(1.,0.,0.));
#34300=DIRECTION('center_axis',(0.,0.,1.));
#34301=DIRECTION('ref_axis',(1.,0.,0.));
#34302=DIRECTION('center_axis',(0.,0.,1.));
#34303=DIRECTION('ref_axis',(1.,0.,0.));
#34304=DIRECTION('center_axis',(0.,0.,1.));
#34305=DIRECTION('ref_axis',(1.,-5.87495706799284E-15,0.));
#34306=DIRECTION('center_axis',(0.,0.,-1.));
#34307=DIRECTION('ref_axis',(1.,-5.87495706799284E-15,0.));
#34308=DIRECTION('center_axis',(0.,0.,1.));
#34309=DIRECTION('ref_axis',(-0.944006790271089,-0.329926021892902,0.));
#34310=DIRECTION('center_axis',(0.,0.,1.));
#34311=DIRECTION('ref_axis',(1.,0.,0.));
#34312=DIRECTION('center_axis',(0.,0.,-1.));
#34313=DIRECTION('ref_axis',(-1.,0.,0.));
#34314=DIRECTION('center_axis',(0.,0.,1.));
#34315=DIRECTION('ref_axis',(1.,0.,0.));
#34316=DIRECTION('center_axis',(0.,0.,1.));
#34317=DIRECTION('ref_axis',(1.,0.,0.));
#34318=DIRECTION('center_axis',(0.,0.,1.));
#34319=DIRECTION('ref_axis',(1.,0.,0.));
#34320=DIRECTION('',(0.707106781186568,8.65956056235518E-17,-0.707106781186527));
#34321=DIRECTION('center_axis',(0.,0.,1.));
#34322=DIRECTION('ref_axis',(1.,0.,0.));
#34323=DIRECTION('center_axis',(0.,0.,1.));
#34324=DIRECTION('ref_axis',(1.,0.,0.));
#34325=DIRECTION('',(0.,0.,-1.));
#34326=DIRECTION('center_axis',(0.,0.,-1.));
#34327=DIRECTION('ref_axis',(1.,0.,0.));
#34328=DIRECTION('center_axis',(0.,0.,1.));
#34329=DIRECTION('ref_axis',(1.,0.,0.));
#34330=DIRECTION('',(-0.707106781186534,-8.65956056235477E-17,-0.707106781186561));
#34331=DIRECTION('center_axis',(0.,0.,1.));
#34332=DIRECTION('ref_axis',(1.,0.,0.));
#34333=DIRECTION('center_axis',(0.,0.,-1.));
#34334=DIRECTION('ref_axis',(-1.,0.,0.));
#34335=DIRECTION('center_axis',(0.,0.,1.));
#34336=DIRECTION('ref_axis',(1.,0.,0.));
#34337=DIRECTION('center_axis',(0.,0.,1.));
#34338=DIRECTION('ref_axis',(1.,0.,0.));
#34339=DIRECTION('center_axis',(0.,0.,1.));
#34340=DIRECTION('ref_axis',(1.,0.,0.));
#34341=DIRECTION('',(0.707106781186568,8.65956056235518E-17,-0.707106781186527));
#34342=DIRECTION('center_axis',(0.,0.,1.));
#34343=DIRECTION('ref_axis',(1.,0.,0.));
#34344=DIRECTION('center_axis',(0.,0.,1.));
#34345=DIRECTION('ref_axis',(1.,0.,0.));
#44018=CARTESIAN_POINT('',(0.,0.,0.));
#44019=CARTESIAN_POINT('Origin',(0.,0.,131.75));
#44020=CARTESIAN_POINT('',(-1.48662474598514,6.70630482219048E-6,131.11245853209));
#44021=CARTESIAN_POINT('',(-1.4866687345303,-8.57105652977442E-7,131.06254146791));
#44022=CARTESIAN_POINT('',(-1.486725,-1.82071301246235E-16,131.75));
#44023=CARTESIAN_POINT('',(0.644080091015134,1.33993887967327,131.));
#44024=CARTESIAN_POINT('Ctrl Pts',(-1.48662474598514,6.70630482219048E-6,
131.11245853209));
#44025=CARTESIAN_POINT('Ctrl Pts',(-1.48664238717497,0.112082357541715,
131.10826015708));
#44026=CARTESIAN_POINT('Ctrl Pts',(-1.47411630956215,0.224154129411391,
131.104061782071));
#44027=CARTESIAN_POINT('Ctrl Pts',(-1.44900147170679,0.333329954091576,
131.099863407061));
#44028=CARTESIAN_POINT('Ctrl Pts',(-1.39531127956612,0.566724692212197,
131.090888172491));
#44029=CARTESIAN_POINT('Ctrl Pts',(-1.28408873642491,0.786884556765062,
131.081912937921));
#44030=CARTESIAN_POINT('Ctrl Pts',(-1.12807594748543,0.968587090660957,
131.072937703351));
#44031=CARTESIAN_POINT('Ctrl Pts',(-0.972063158545943,1.15028962455685,
131.063962468781));
#44032=CARTESIAN_POINT('Ctrl Pts',(-0.771260123808195,1.29353482779577,
131.054987234211));
#44033=CARTESIAN_POINT('Ctrl Pts',(-0.548672624156139,1.38191112458742,
131.046011999641));
#44034=CARTESIAN_POINT('Ctrl Pts',(-0.326085124504082,1.47028742137907,
131.03703676507));
#44035=CARTESIAN_POINT('Ctrl Pts',(-0.0817131599377159,1.50379481172344,
131.0280615305));
#44036=CARTESIAN_POINT('Ctrl Pts',(0.156447623458401,1.47859617596776,131.01908629593));
#44037=CARTESIAN_POINT('Ctrl Pts',(0.325267990783618,1.46073411285348,131.012724197287));
#44038=CARTESIAN_POINT('Ctrl Pts',(0.490967432775488,1.41337409773075,131.006362098643));
#44039=CARTESIAN_POINT('Ctrl Pts',(0.644080091015134,1.33993887967327,131.));
#44040=CARTESIAN_POINT('',(-0.644068464422626,1.33997277538063,131.));
#44041=CARTESIAN_POINT('Origin',(0.,0.,131.));
#44042=CARTESIAN_POINT('Ctrl Pts',(-0.644068464422466,1.33997277538071,
131.));
#44043=CARTESIAN_POINT('Ctrl Pts',(-0.859968943773443,1.23619851014301,
131.00897523457));
#44044=CARTESIAN_POINT('Ctrl Pts',(-1.05021748697928,1.07929218747651,131.01795046914));
#44045=CARTESIAN_POINT('Ctrl Pts',(-1.19311574373449,0.887131970323545,
131.02692570371));
#44046=CARTESIAN_POINT('Ctrl Pts',(-1.33601400048969,0.694971753170582,
131.03590093828));
#44047=CARTESIAN_POINT('Ctrl Pts',(-1.43156197079426,0.467557641531158,
131.044876172851));
#44048=CARTESIAN_POINT('Ctrl Pts',(-1.46877946004656,0.230978828954324,
131.053851407421));
#44049=CARTESIAN_POINT('Ctrl Pts',(-1.48079111390487,0.154624865697416,
131.056748094251));
#44050=CARTESIAN_POINT('Ctrl Pts',(-1.48672691792441,0.0773162841053159,
131.05964478108));
#44051=CARTESIAN_POINT('Ctrl Pts',(-1.4866687345303,-8.57105652977442E-7,
131.06254146791));
#44052=CARTESIAN_POINT('Origin',(0.,0.,131.75));
#44053=CARTESIAN_POINT('',(-1.48662467006137,6.54543500555605E-6,131.46245853209));
#44054=CARTESIAN_POINT('',(-1.48667651937189,2.89412199965503E-5,131.41254146791));
#44055=CARTESIAN_POINT('',(-1.486725,-1.82071301246235E-16,131.75));
#44056=CARTESIAN_POINT('Ctrl Pts',(-1.48662467006137,6.54543500555605E-6,
131.46245853209));
#44057=CARTESIAN_POINT('Ctrl Pts',(-1.48664293141312,0.111778251545966,
131.458271539825));
#44058=CARTESIAN_POINT('Ctrl Pts',(-1.47418526351766,0.22354594941412,131.454084547561));
#44059=CARTESIAN_POINT('Ctrl Pts',(-1.44920521898838,0.332441071167058,
131.449897555296));
#44060=CARTESIAN_POINT('Ctrl Pts',(-1.39565800775678,0.565868600880252,
131.440922320726));
#44061=CARTESIAN_POINT('Ctrl Pts',(-1.28457023968935,0.786096589160032,
131.431947086156));
#44062=CARTESIAN_POINT('Ctrl Pts',(-1.12866878379445,0.967894420568027,
131.422971851586));
#44063=CARTESIAN_POINT('Ctrl Pts',(-0.972767327899546,1.14969225197602,
131.413996617016));
#44064=CARTESIAN_POINT('Ctrl Pts',(-0.772052184177181,1.29305992651223,
131.405021382445));
#44065=CARTESIAN_POINT('Ctrl Pts',(-0.549518461659608,1.38157239901168,
131.396046147875));
#44066=CARTESIAN_POINT('Ctrl Pts',(-0.326984739142031,1.47008487151113,
131.387070913305));
#44067=CARTESIAN_POINT('Ctrl Pts',(-0.0826324378292454,1.50374214197381,
131.378095678735));
#44068=CARTESIAN_POINT('Ctrl Pts',(0.155544003393841,1.47868823524661,131.369120444165));
#44069=CARTESIAN_POINT('Ctrl Pts',(0.393720444616925,1.45363432851941,131.360145209595));
#44070=CARTESIAN_POINT('Ctrl Pts',(0.62572102575031,1.36986924460234,131.351169975025));
#44071=CARTESIAN_POINT('Ctrl Pts',(0.824966393821326,1.23698960503629,131.342194740455));
#44072=CARTESIAN_POINT('Ctrl Pts',(1.02421176189234,1.10410996547024,131.333219505884));
#44073=CARTESIAN_POINT('Ctrl Pts',(1.19070191690099,0.922115770255228,131.324244271314));
#44074=CARTESIAN_POINT('Ctrl Pts',(1.30536276582783,0.711857346200688,131.315269036744));
#44075=CARTESIAN_POINT('Ctrl Pts',(1.42002361475467,0.501598922146148,131.306293802174));
#44076=CARTESIAN_POINT('Ctrl Pts',(1.4828551575997,0.263076269252084,131.297318567604));
#44077=CARTESIAN_POINT('Ctrl Pts',(1.48665904299347,0.0236159482411607,
131.288343333034));
#44078=CARTESIAN_POINT('Ctrl Pts',(1.49046292838724,-0.215844372769763,
131.279368098464));
#44079=CARTESIAN_POINT('Ctrl Pts',(1.43523915632975,-0.456242361897546,
131.270392863894));
#44080=CARTESIAN_POINT('Ctrl Pts',(1.32731448618016,-0.670036610261909,
131.261417629323));
#44081=CARTESIAN_POINT('Ctrl Pts',(1.21938981603057,-0.883830858626271,
131.252442394753));
#44082=CARTESIAN_POINT('Ctrl Pts',(1.05876424778888,-1.07102136622721,131.243467160183));
#44083=CARTESIAN_POINT('Ctrl Pts',(0.863839993987138,-1.21016248254433,
131.234491925613));
#44084=CARTESIAN_POINT('Ctrl Pts',(0.668915740185388,-1.34930359886145,
131.225516691043));
#44085=CARTESIAN_POINT('Ctrl Pts',(0.439692800823575,-1.44039532389473,
131.216541456473));
#44086=CARTESIAN_POINT('Ctrl Pts',(0.202432300225987,-1.47300165684166,
131.207566221903));
#44087=CARTESIAN_POINT('Ctrl Pts',(-0.0348282003715965,-1.5056079897886,
131.198590987333));
#44088=CARTESIAN_POINT('Ctrl Pts',(-0.280126262204957,-1.47972893064917,
131.189615752763));
#44089=CARTESIAN_POINT('Ctrl Pts',(-0.505359087071109,-1.39832932086742,
131.180640518192));
#44090=CARTESIAN_POINT('Ctrl Pts',(-0.730591911937262,-1.31692971108566,
131.171665283622));
#44091=CARTESIAN_POINT('Ctrl Pts',(-0.935759499836208,-1.18000955066158,
131.162690049052));
#44092=CARTESIAN_POINT('Ctrl Pts',(-1.09735667018443,-1.00325523997758,
131.153714814482));
#44093=CARTESIAN_POINT('Ctrl Pts',(-1.25895384053266,-0.826500929293591,
131.144739579912));
#44094=CARTESIAN_POINT('Ctrl Pts',(-1.37698059333016,-0.609912468349694,
131.135764345342));
#44095=CARTESIAN_POINT('Ctrl Pts',(-1.43791504915886,-0.378303432033558,
131.126789110772));
#44096=CARTESIAN_POINT('Ctrl Pts',(-1.47034599406822,-0.255034916788333,
131.122012251211));
#44097=CARTESIAN_POINT('Ctrl Pts',(-1.48660467405586,-0.127511594203174,
131.117235391651));
#44098=CARTESIAN_POINT('Ctrl Pts',(-1.48662474598514,6.70630482219048E-6,
131.11245853209));
#44099=CARTESIAN_POINT('Ctrl Pts',(-1.4866687345303,-8.57105652977442E-7,
131.06254146791));
#44100=CARTESIAN_POINT('Ctrl Pts',(-1.48654663968209,-0.162246885628005,
131.06862001565));
#44101=CARTESIAN_POINT('Ctrl Pts',(-1.46003010793999,-0.324530606308262,
131.074698563391));
#44102=CARTESIAN_POINT('Ctrl Pts',(-1.40787558798148,-0.478109975852054,
131.080777111131));
#44103=CARTESIAN_POINT('Ctrl Pts',(-1.33086721846408,-0.704876454567354,
131.089752345701));
#44104=CARTESIAN_POINT('Ctrl Pts',(-1.19796347122924,-0.91266589848371,
131.098727580271));
#44105=CARTESIAN_POINT('Ctrl Pts',(-1.02438398444855,-1.07766566984475,
131.107702814842));
#44106=CARTESIAN_POINT('Ctrl Pts',(-0.85080449766787,-1.2426654412058,131.116678049412));
#44107=CARTESIAN_POINT('Ctrl Pts',(-0.636549271341341,-1.36487554001152,
131.125653283982));
#44108=CARTESIAN_POINT('Ctrl Pts',(-0.406167987067542,-1.43029720218641,
131.134628518552));
#44109=CARTESIAN_POINT('Ctrl Pts',(-0.175786702793742,-1.49571886436129,
131.143603753122));
#44110=CARTESIAN_POINT('Ctrl Pts',(0.0707206394273271,-1.50435208990532,
131.152578987692));
#44111=CARTESIAN_POINT('Ctrl Pts',(0.30511402383943,-1.45520632418145,131.161554222262));
#44112=CARTESIAN_POINT('Ctrl Pts',(0.539507408251534,-1.40606055845758,
131.170529456832));
#44113=CARTESIAN_POINT('Ctrl Pts',(0.761786834854671,-1.2991358014658,131.179504691402));
#44114=CARTESIAN_POINT('Ctrl Pts',(0.946485973897794,-1.14668243377515,
131.188479925973));
#44115=CARTESIAN_POINT('Ctrl Pts',(1.13118511294092,-0.994229066084504,
131.197455160543));
#44116=CARTESIAN_POINT('Ctrl Pts',(1.27830396442402,-0.796247087694984,
131.206430395113));
#44117=CARTESIAN_POINT('Ctrl Pts',(1.37098798792177,-0.57541816644418,131.215405629683));
#44118=CARTESIAN_POINT('Ctrl Pts',(1.46367201141952,-0.354589245193374,
131.224380864253));
#44119=CARTESIAN_POINT('Ctrl Pts',(1.5019212069319,-0.11091338108128,131.233356098823));
#44120=CARTESIAN_POINT('Ctrl Pts',(1.48135337845442,0.127692398802491,131.242331333393));
#44121=CARTESIAN_POINT('Ctrl Pts',(1.46078554997695,0.366298178686261,131.251306567963));
#44122=CARTESIAN_POINT('Ctrl Pts',(1.38140069750961,0.599833874341709,131.260281802533));
#44123=CARTESIAN_POINT('Ctrl Pts',(1.25229366895348,0.801544328040148,131.269257037104));
#44124=CARTESIAN_POINT('Ctrl Pts',(1.12318664039736,1.00325478173859,131.278232271674));
#44125=CARTESIAN_POINT('Ctrl Pts',(0.944357435752443,1.17313999348001,131.287207506244));
#44126=CARTESIAN_POINT('Ctrl Pts',(0.736293752205015,1.29173689729788,131.296182740814));
#44127=CARTESIAN_POINT('Ctrl Pts',(0.528230068657587,1.41033380111575,131.305157975384));
#44128=CARTESIAN_POINT('Ctrl Pts',(0.290931906207645,1.47764239701006,131.314133209954));
#44129=CARTESIAN_POINT('Ctrl Pts',(0.0515855500820499,1.48595143028722,
131.323108444524));
#44130=CARTESIAN_POINT('Ctrl Pts',(-0.187760806043545,1.49426046356437,
131.332083679094));
#44131=CARTESIAN_POINT('Ctrl Pts',(-0.429155355844794,1.44356993422436,
131.341058913665));
#44132=CARTESIAN_POINT('Ctrl Pts',(-0.64494252417023,1.33968724516187,131.350034148235));
#44133=CARTESIAN_POINT('Ctrl Pts',(-0.860729692495666,1.23580455609938,
131.359009382805));
#44134=CARTESIAN_POINT('Ctrl Pts',(-1.05090947934529,1.07872970731441,131.367984617375));
#44135=CARTESIAN_POINT('Ctrl Pts',(-1.1936937662667,0.8864581217929,131.376959851945));
#44136=CARTESIAN_POINT('Ctrl Pts',(-1.33647805318811,0.694186536271395,
131.385935086515));
#44137=CARTESIAN_POINT('Ctrl Pts',(-1.4318668401813,0.466718214013358,131.394910321085));
#44138=CARTESIAN_POINT('Ctrl Pts',(-1.46893182730532,0.230113265328173,
131.403885555655));
#44139=CARTESIAN_POINT('Ctrl Pts',(-1.48084725502128,0.154050938532649,
131.40677085974));
#44140=CARTESIAN_POINT('Ctrl Pts',(-1.48673518054972,0.0770443825219525,
131.409656163825));
#44141=CARTESIAN_POINT('Ctrl Pts',(-1.48667651937189,2.89412199965503E-5,
131.41254146791));
#44142=CARTESIAN_POINT('Origin',(0.,0.,131.75));
#44143=CARTESIAN_POINT('',(-1.48662482583238,6.78982369262116E-6,131.81245853209));
#44144=CARTESIAN_POINT('',(-1.48667723510369,2.90658880924576E-5,131.76254146791));
#44145=CARTESIAN_POINT('',(-1.486725,-1.82071301246235E-16,131.75));
#44146=CARTESIAN_POINT('Ctrl Pts',(-1.48662482583238,6.78982369262116E-6,
131.81245853209));
#44147=CARTESIAN_POINT('Ctrl Pts',(-1.48664372040861,0.111474600180848,
131.80828292257));
#44148=CARTESIAN_POINT('Ctrl Pts',(-1.47425429712656,0.222938274562959,
131.80410731305));
#44149=CARTESIAN_POINT('Ctrl Pts',(-1.44940874218647,0.331552605768891,
131.799931703531));
#44150=CARTESIAN_POINT('Ctrl Pts',(-1.39600463853288,0.565012917521814,
131.790956468961));
#44151=CARTESIAN_POINT('Ctrl Pts',(-1.28505189717003,0.785308964263988,
131.78198123439));
#44152=CARTESIAN_POINT('Ctrl Pts',(-1.12926191763864,0.967202333379871,
131.77300599982));
#44153=CARTESIAN_POINT('Ctrl Pts',(-0.973471938107258,1.14909570249575,
131.76403076525));
#44154=CARTESIAN_POINT('Ctrl Pts',(-0.772844720407338,1.29258639398535,
131.75505553068));
#44155=CARTESIAN_POINT('Ctrl Pts',(-0.550365300254005,1.38123526909931,
131.74608029611));
#44156=CARTESIAN_POINT('Ctrl Pts',(-0.327885880100671,1.46988414421327,
131.73710506154));
#44157=CARTESIAN_POINT('Ctrl Pts',(-0.0835542574939237,1.5036912029516,
131.72812982697));
#44158=CARTESIAN_POINT('Ctrl Pts',(0.15463749781462,1.47878330954827,131.7191545924));
#44159=CARTESIAN_POINT('Ctrl Pts',(0.392829253123164,1.45387541614494,131.710179357829));
#44160=CARTESIAN_POINT('Ctrl Pts',(0.624881141133504,1.37025257059994,131.701204123259));
#44161=CARTESIAN_POINT('Ctrl Pts',(0.824207930814637,1.23749509862122,131.692228888689));
#44162=CARTESIAN_POINT('Ctrl Pts',(1.02353472049577,1.1047376266425,131.683253654119));
#44163=CARTESIAN_POINT('Ctrl Pts',(1.1901364118477,0.922845528230054,131.674278419549));
#44164=CARTESIAN_POINT('Ctrl Pts',(1.30492613385756,0.712657433487139,131.665303184979));
#44165=CARTESIAN_POINT('Ctrl Pts',(1.41971585586741,0.502469338744224,131.656327950409));
#44166=CARTESIAN_POINT('Ctrl Pts',(1.4826936085352,0.263985247670841,131.647352715839));
#44167=CARTESIAN_POINT('Ctrl Pts',(1.48664428958854,0.0245273023653047,
131.638377481268));
#44168=CARTESIAN_POINT('Ctrl Pts',(1.49059497064187,-0.214930642940232,
131.629402246698));
#44169=CARTESIAN_POINT('Ctrl Pts',(1.43551858008075,-0.455362442477921,
131.620427012128));
#44170=CARTESIAN_POINT('Ctrl Pts',(1.32772499359706,-0.669222813196063,
131.611451777558));
#44171=CARTESIAN_POINT('Ctrl Pts',(1.21993140711338,-0.883083183914204,
131.602476542988));
#44172=CARTESIAN_POINT('Ctrl Pts',(1.05942062470712,-1.0703721258128,131.593501308418));
#44173=CARTESIAN_POINT('Ctrl Pts',(0.864581706987901,-1.20963271461242,
131.584526073848));
#44174=CARTESIAN_POINT('Ctrl Pts',(0.669742789268677,-1.34889330341204,
131.575550839278));
#44175=CARTESIAN_POINT('Ctrl Pts',(0.440575736236482,-1.44012553911268,
131.566575604708));
#44176=CARTESIAN_POINT('Ctrl Pts',(0.203335275236014,-1.47287731945189,
131.557600370137));
#44177=CARTESIAN_POINT('Ctrl Pts',(-0.033905185764455,-1.50562909979111,
131.548625135567));
#44178=CARTESIAN_POINT('Ctrl Pts',(-0.279219054733197,-1.47990042476888,
131.539649900997));
#44179=CARTESIAN_POINT('Ctrl Pts',(-0.504501729990859,-1.39863892293247,
131.530674666427));
#44180=CARTESIAN_POINT('Ctrl Pts',(-0.72978440524852,-1.31737742109606,
131.521699431857));
#44181=CARTESIAN_POINT('Ctrl Pts',(-0.9350358867951,-1.18058309244548,131.512724197287));
#44182=CARTESIAN_POINT('Ctrl Pts',(-1.09674135601336,-1.00392790096093,
131.503748962717));
#44183=CARTESIAN_POINT('Ctrl Pts',(-1.25844682523162,-0.827272709476379,
131.494773728147));
#44184=CARTESIAN_POINT('Ctrl Pts',(-1.37660628212157,-0.610756655157868,
131.485798493576));
#44185=CARTESIAN_POINT('Ctrl Pts',(-1.43768268336866,-0.379185092425305,
131.476823259006));
#44186=CARTESIAN_POINT('Ctrl Pts',(-1.4702666349111,-0.255642833473939,
131.472035016701));
#44187=CARTESIAN_POINT('Ctrl Pts',(-1.48660378638844,-0.127815522989732,
131.467246774395));
#44188=CARTESIAN_POINT('Ctrl Pts',(-1.48662467006137,6.54543500555605E-6,
131.46245853209));
#44189=CARTESIAN_POINT('Ctrl Pts',(-1.48667651937189,2.89412199965503E-5,
131.41254146791));
#44190=CARTESIAN_POINT('Ctrl Pts',(-1.48655270486754,-0.162525392751979,
131.418631398395));
#44191=CARTESIAN_POINT('Ctrl Pts',(-1.45993722594017,-0.325119310129694,
131.424721328881));
#44192=CARTESIAN_POINT('Ctrl Pts',(-1.40759092349875,-0.478957857091241,
131.430811259366));
#44193=CARTESIAN_POINT('Ctrl Pts',(-1.33044384531333,-0.705682455713139,
131.439786493936));
#44194=CARTESIAN_POINT('Ctrl Pts',(-1.19740850168767,-0.913390077844603,
131.448761728506));
#44195=CARTESIAN_POINT('Ctrl Pts',(-1.02372620542085,-1.07828451499433,
131.457736963076));
#44196=CARTESIAN_POINT('Ctrl Pts',(-0.850043909154037,-1.24317895214406,
131.466712197646));
#44197=CARTESIAN_POINT('Ctrl Pts',(-0.63571466024607,-1.36526020431205,
131.475687432216));
#44198=CARTESIAN_POINT('Ctrl Pts',(-0.405293279741281,-1.43054192405704,
131.484662666787));
#44199=CARTESIAN_POINT('Ctrl Pts',(-0.174871899236492,-1.49582364380202,
131.493637901357));
#44200=CARTESIAN_POINT('Ctrl Pts',(0.0716416128651196,-1.50430583112399,
131.502613135927));
#44201=CARTESIAN_POINT('Ctrl Pts',(0.306005216640002,-1.45501671668872,
131.511588370497));
#44202=CARTESIAN_POINT('Ctrl Pts',(0.540368820414884,-1.40572760225345,
131.520563605067));
#44203=CARTESIAN_POINT('Ctrl Pts',(0.762582515863036,-1.29866718606095,
131.529538839637));
#44204=CARTESIAN_POINT('Ctrl Pts',(0.947188193250521,-1.14610093991915,
131.538514074207));
#44205=CARTESIAN_POINT('Ctrl Pts',(1.13179387063801,-0.993534693777357,
131.547489308777));
#44206=CARTESIAN_POINT('Ctrl Pts',(1.27879152996482,-0.795462617686266,
131.556464543347));
#44207=CARTESIAN_POINT('Ctrl Pts',(1.37134025357767,-0.574577015287615,
131.565439777918));
#44208=CARTESIAN_POINT('Ctrl Pts',(1.46388897719051,-0.353691412888964,
131.574415012488));
#44209=CARTESIAN_POINT('Ctrl Pts',(1.50198876508937,-0.109992284182755,
131.583390247058));
#44210=CARTESIAN_POINT('Ctrl Pts',(1.48127468117422,0.128600763314322,131.592365481628));
#44211=CARTESIAN_POINT('Ctrl Pts',(1.46056059725906,0.367193810811399,131.601340716198));
#44212=CARTESIAN_POINT('Ctrl Pts',(1.38103264152987,0.600680777099344,131.610315950768));
#44213=CARTESIAN_POINT('Ctrl Pts',(1.25180200499627,0.802312020128169,131.619291185338));
#44214=CARTESIAN_POINT('Ctrl Pts',(1.12257136846268,1.00394326315699,131.628266419908));
#44215=CARTESIAN_POINT('Ctrl Pts',(0.943638051124673,1.1737187829267,131.637241654478));
#44216=CARTESIAN_POINT('Ctrl Pts',(0.73550170769923,1.29218809594964,131.646216889049));
#44217=CARTESIAN_POINT('Ctrl Pts',(0.527365364273789,1.41065740897258,131.655192123619));
#44218=CARTESIAN_POINT('Ctrl Pts',(0.29002599476091,1.47782051524875,131.664167358189));
#44219=CARTESIAN_POINT('Ctrl Pts',(0.0506745952140745,1.48598281374583,
131.673142592759));
#44220=CARTESIAN_POINT('Ctrl Pts',(-0.188676804332765,1.4941451122429,131.682117827329));
#44221=CARTESIAN_POINT('Ctrl Pts',(-0.430040233913561,1.44330660296088,
131.691093061899));
#44222=CARTESIAN_POINT('Ctrl Pts',(-0.645763677451843,1.3392916449525,131.700068296469));
#44223=CARTESIAN_POINT('Ctrl Pts',(-0.861487120990125,1.23527668694413,
131.709043531039));
#44224=CARTESIAN_POINT('Ctrl Pts',(-1.05157057848589,1.07808528020941,131.71801876561));
#44225=CARTESIAN_POINT('Ctrl Pts',(-1.19423696949397,0.885726198130794,
131.72699400018));
#44226=CARTESIAN_POINT('Ctrl Pts',(-1.33690336050205,0.693367116052179,
131.73596923475));
#44227=CARTESIAN_POINT('Ctrl Pts',(-1.43215268502245,0.465840358629668,
131.74494446932));
#44228=CARTESIAN_POINT('Ctrl Pts',(-1.46907261943811,0.22921273128206,131.75391970389));
#44229=CARTESIAN_POINT('Ctrl Pts',(-1.48089459317689,0.153443214335519,
131.75679362523));
#44230=CARTESIAN_POINT('Ctrl Pts',(-1.4867359556546,0.0767405697656338,
131.75966754657));
#44231=CARTESIAN_POINT('Ctrl Pts',(-1.48667723510369,2.90658880924576E-5,
131.76254146791));
#44232=CARTESIAN_POINT('Origin',(0.,0.,131.75));
#44233=CARTESIAN_POINT('',(-1.48662495810528,7.0294833549589E-6,132.16245853209));
#44234=CARTESIAN_POINT('',(-1.48667795283619,2.91850407830213E-5,132.11254146791));
#44235=CARTESIAN_POINT('',(-1.486725,-1.82071301246235E-16,131.75));
#44236=CARTESIAN_POINT('Ctrl Pts',(-1.48662495810528,7.0294833549589E-6,
132.16245853209));
#44237=CARTESIAN_POINT('Ctrl Pts',(-1.48664448474531,0.111170943043426,
132.158294305315));
#44238=CARTESIAN_POINT('Ctrl Pts',(-1.47432311674833,0.222330594316862,
132.15413007854));
#44239=CARTESIAN_POINT('Ctrl Pts',(-1.44961170010174,0.330664011192151,
132.149965851765));
#44240=CARTESIAN_POINT('Ctrl Pts',(-1.3963507292296,0.564157017408393,132.140990617195));
#44241=CARTESIAN_POINT('Ctrl Pts',(-1.28553305875945,0.784521041741841,
132.132015382625));
#44242=CARTESIAN_POINT('Ctrl Pts',(-1.12985461636972,0.966509881058128,
132.123040148055));
#44243=CARTESIAN_POINT('Ctrl Pts',(-0.974176173979993,1.14849872037442,
132.114064913485));
#44244=CARTESIAN_POINT('Ctrl Pts',(-0.773636959670693,1.29211237467355,
132.105089678915));
#44245=CARTESIAN_POINT('Ctrl Pts',(-0.551211926840969,1.38089761924403,
132.096114444345));
#44246=CARTESIAN_POINT('Ctrl Pts',(-0.328786894011251,1.46968286381452,
132.087139209774));
#44247=CARTESIAN_POINT('Ctrl Pts',(-0.0844760426611109,1.50363969865637,
132.078163975204));
#44248=CARTESIAN_POINT('Ctrl Pts',(0.153730936532854,1.47887782825435,132.069188740634));
#44249=CARTESIAN_POINT('Ctrl Pts',(0.391937915726826,1.45411595785233,132.060213506064));
#44250=CARTESIAN_POINT('Ctrl Pts',(0.624041022764623,1.37063538220644,132.051238271494));
#44251=CARTESIAN_POINT('Ctrl Pts',(0.823449158655619,1.23800012803382,132.042263036924));
#44252=CARTESIAN_POINT('Ctrl Pts',(1.02285729454661,1.1053648738612,132.033287802354));
#44253=CARTESIAN_POINT('Ctrl Pts',(1.1895704592908,0.92357494116184,132.024312567784));
#44254=CARTESIAN_POINT('Ctrl Pts',(1.30448901068812,0.713457255231484,132.015337333214));
#44255=CARTESIAN_POINT('Ctrl Pts',(1.41940756208544,0.503339569301124,132.006362098643));
#44256=CARTESIAN_POINT('Ctrl Pts',(1.48253150013589,0.264894130139772,131.997386864073));
#44257=CARTESIAN_POINT('Ctrl Pts',(1.48662897469899,0.025438651714869,131.988411629503));
#44258=CARTESIAN_POINT('Ctrl Pts',(1.49072644926209,-0.214016826710032,
131.979436394933));
#44259=CARTESIAN_POINT('Ctrl Pts',(1.43579746033784,-0.454482344398475,
131.970461160363));
#44260=CARTESIAN_POINT('Ctrl Pts',(1.32813499638598,-0.668408755368728,
131.961485925793));
#44261=CARTESIAN_POINT('Ctrl Pts',(1.22047253243412,-0.882335166338984,
131.952510691223));
#44262=CARTESIAN_POINT('Ctrl Pts',(1.06007659345464,-1.06972247059105,131.943535456653));
#44263=CARTESIAN_POINT('Ctrl Pts',(0.865323082913764,-1.20910247486244,
131.934560222082));
#44264=CARTESIAN_POINT('Ctrl Pts',(0.670569572372892,-1.34848247913384,
131.925584987512));
#44265=CARTESIAN_POINT('Ctrl Pts',(0.441458490270625,-1.43985518342455,
131.916609752942));
#44266=CARTESIAN_POINT('Ctrl Pts',(0.20423815158461,-1.4727523925674,131.907634518372));
#44267=CARTESIAN_POINT('Ctrl Pts',(-0.0329821871014054,-1.50564960171024,
131.898659283802));
#44268=CARTESIAN_POINT('Ctrl Pts',(-0.27831178237117,-1.4800713157052,131.889684049232));
#44269=CARTESIAN_POINT('Ctrl Pts',(-0.50364423084838,-1.39894793364549,
131.880708814662));
#44270=CARTESIAN_POINT('Ctrl Pts',(-0.728976679325591,-1.31782455158578,
131.871733580092));
#44271=CARTESIAN_POINT('Ctrl Pts',(-0.934311981010247,-1.18115607347139,
131.862758345521));
#44272=CARTESIAN_POINT('Ctrl Pts',(-1.09612571435821,-1.0046000451066,131.853783110951));
#44273=CARTESIAN_POINT('Ctrl Pts',(-1.25793944770617,-0.828044016741798,
131.844807876381));
#44274=CARTESIAN_POINT('Ctrl Pts',(-1.37623161271745,-0.611600438126588,
131.835832641811));
#44275=CARTESIAN_POINT('Ctrl Pts',(-1.43744996225092,-0.380066360437146,
131.826857407241));
#44276=CARTESIAN_POINT('Ctrl Pts',(-1.47018728200171,-0.256250458958468,
131.822057782191));
#44277=CARTESIAN_POINT('Ctrl Pts',(-1.48660310759437,-0.12811910230264,
131.81725815714));
#44278=CARTESIAN_POINT('Ctrl Pts',(-1.48662482583238,6.78982369262116E-6,
131.81245853209));
#44279=CARTESIAN_POINT('Ctrl Pts',(-1.48667723510369,2.90658880924576E-5,
131.76254146791));
#44280=CARTESIAN_POINT('Ctrl Pts',(-1.48655257181903,-0.162828875630418,
131.76864278114));
#44281=CARTESIAN_POINT('Ctrl Pts',(-1.45983566302084,-0.325726746906379,
131.77474409437));
#44282=CARTESIAN_POINT('Ctrl Pts',(-1.4072970457122,-0.479820656595399,
131.7808454076));
#44283=CARTESIAN_POINT('Ctrl Pts',(-1.3300109932597,-0.706497919852542,
131.789820642171));
#44284=CARTESIAN_POINT('Ctrl Pts',(-1.19684834404377,-0.914123949094121,
131.798795876741));
#44285=CARTESIAN_POINT('Ctrl Pts',(-1.02306499546073,-1.07891188353324,
131.807771111311));
#44286=CARTESIAN_POINT('Ctrl Pts',(-0.849281646877681,-1.24369981797236,
131.816746345881));
#44287=CARTESIAN_POINT('Ctrl Pts',(-0.634877598927511,-1.36564965760903,
131.825721580451));
#44288=CARTESIAN_POINT('Ctrl Pts',(-0.404416242141579,-1.43079011055361,
131.834696815021));
#44289=CARTESIAN_POINT('Ctrl Pts',(-0.173954885355643,-1.49593056349819,
131.843672049591));
#44290=CARTESIAN_POINT('Ctrl Pts',(0.072563780266055,-1.50426162975068,
131.852647284161));
#44291=CARTESIAN_POINT('Ctrl Pts',(0.306897124442854,-1.4548288532928,131.861622518732));
#44292=CARTESIAN_POINT('Ctrl Pts',(0.54123046861965,-1.40539607683492,131.870597753302));
#44293=CARTESIAN_POINT('Ctrl Pts',(0.763378491351546,-1.29819945766667,
131.879572987872));
#44294=CARTESIAN_POINT('Ctrl Pts',(0.947890606745602,-1.14552007184721,
131.888548222442));
#44295=CARTESIAN_POINT('Ctrl Pts',(1.13240272213966,-0.992840686027748,
131.897523457012));
#44296=CARTESIAN_POINT('Ctrl Pts',(1.27927893019587,-0.794678533557074,
131.906498691582));
#44297=CARTESIAN_POINT('Ctrl Pts',(1.37169222744692,-0.573736237758631,
131.915473926152));
#44298=CARTESIAN_POINT('Ctrl Pts',(1.46410552469796,-0.352793941960185,
131.924449160722));
#44299=CARTESIAN_POINT('Ctrl Pts',(1.50205591114383,-0.109071502833969,
131.933424395292));
#44300=CARTESIAN_POINT('Ctrl Pts',(1.48119556699242,0.129508801515888,131.942399629863));
#44301=CARTESIAN_POINT('Ctrl Pts',(1.46033522284101,0.368089105865746,131.951374864433));
#44302=CARTESIAN_POINT('Ctrl Pts',(1.38066414809232,0.601527275439246,131.960350099003));
#44303=CARTESIAN_POINT('Ctrl Pts',(1.25130993031637,0.803079258625255,131.969325333573));
#44304=CARTESIAN_POINT('Ctrl Pts',(1.12195571254041,1.00463124181126,131.978300568143));
#44305=CARTESIAN_POINT('Ctrl Pts',(0.942918351737199,1.17429703860978,131.987275802713));
#44306=CARTESIAN_POINT('Ctrl Pts',(0.734709422453624,1.29263873604062,131.996251037283));
#44307=CARTESIAN_POINT('Ctrl Pts',(0.526500493170048,1.41098043347147,132.005226271853));
#44308=CARTESIAN_POINT('Ctrl Pts',(0.289119995406113,1.47799803153465,132.014201506424));
#44309=CARTESIAN_POINT('Ctrl Pts',(0.0497636371096859,1.48601359947829,
132.023176740994));
#44310=CARTESIAN_POINT('Ctrl Pts',(-0.189592721186742,1.49402916742193,
132.032151975564));
#44311=CARTESIAN_POINT('Ctrl Pts',(-0.430924940015661,1.44304270524602,
132.041127210134));
#44312=CARTESIAN_POINT('Ctrl Pts',(-0.646584578996447,1.33889552235537,
132.050102444704));
#44313=CARTESIAN_POINT('Ctrl Pts',(-0.862244217977232,1.23474833946472,
132.059077679274));
#44314=CARTESIAN_POINT('Ctrl Pts',(-1.05223127710988,1.07744043585933,132.068052913844));
#44315=CARTESIAN_POINT('Ctrl Pts',(-1.1947797199153,0.88499393150229,132.077028148414));
#44316=CARTESIAN_POINT('Ctrl Pts',(-1.33732816272071,0.692547427145254,
132.086003382984));
#44317=CARTESIAN_POINT('Ctrl Pts',(-1.43243798919889,0.46496232203658,132.094978617555));
#44318=CARTESIAN_POINT('Ctrl Pts',(-1.46921285748553,0.228312106235572,
132.103953852125));
#44319=CARTESIAN_POINT('Ctrl Pts',(-1.48094174088988,0.152835485432742,
132.10681639072));
#44320=CARTESIAN_POINT('Ctrl Pts',(-1.48673672765572,0.0764367515174225,
132.109678929315));
#44321=CARTESIAN_POINT('Ctrl Pts',(-1.48667795283619,2.91850407830213E-5,
132.11254146791));
#44322=CARTESIAN_POINT('Origin',(0.,0.,131.75));
#44323=CARTESIAN_POINT('',(-1.486725,-1.82071301246235E-16,132.5));
#44324=CARTESIAN_POINT('',(-1.48668131839924,3.04819389219259E-5,132.46254146791));
#44325=CARTESIAN_POINT('',(-1.486725,-1.82071301246235E-16,131.75));
#44326=CARTESIAN_POINT('',(-1.44969557651742,0.329748329868144,132.5));
#44327=CARTESIAN_POINT('Origin',(0.,0.,132.5));
#44328=CARTESIAN_POINT('Ctrl Pts',(-1.44969557651734,0.329748329868494,
132.5));
#44329=CARTESIAN_POINT('Ctrl Pts',(-1.39656552507766,0.563327679862336,
132.49102476543));
#44330=CARTESIAN_POINT('Ctrl Pts',(-1.28592745851384,0.783721236611964,
132.48204953086));
#44331=CARTESIAN_POINT('Ctrl Pts',(-1.1303829541632,0.965796406696618,132.47307429629));
#44332=CARTESIAN_POINT('Ctrl Pts',(-0.974838449812451,1.1478715767814,132.46409906172));
#44333=CARTESIAN_POINT('Ctrl Pts',(-0.774387507674821,1.29162836020115,
132.455123827149));
#44334=CARTESIAN_POINT('Ctrl Pts',(-0.552021890034789,1.38055646740327,
132.446148592579));
#44335=CARTESIAN_POINT('Ctrl Pts',(-0.329656272394756,1.46948457460539,
132.437173358009));
#44336=CARTESIAN_POINT('Ctrl Pts',(-0.0853759792523218,1.50358400558988,
132.428198123439));
#44337=CARTESIAN_POINT('Ctrl Pts',(0.152840964869851,1.47896668523315,132.419222888869));
#44338=CARTESIAN_POINT('Ctrl Pts',(0.39105790899202,1.45434936487643,132.410247654299));
#44339=CARTESIAN_POINT('Ctrl Pts',(0.623211504093927,1.3710152931785,132.401272419729));
#44340=CARTESIAN_POINT('Ctrl Pts',(0.82269945647758,1.23850370981599,132.392297185159));
#44341=CARTESIAN_POINT('Ctrl Pts',(1.02218740886124,1.10599212645348,132.383321950588));
#44342=CARTESIAN_POINT('Ctrl Pts',(1.18900971852664,0.924303031426379,132.374346716018));
#44343=CARTESIAN_POINT('Ctrl Pts',(1.3040557817562,0.714255576485402,132.365371481448));
#44344=CARTESIAN_POINT('Ctrl Pts',(1.41910184498576,0.504208121544427,132.356396246878));
#44345=CARTESIAN_POINT('Ctrl Pts',(1.48237166177948,0.265802306689577,132.347421012308));
#44346=CARTESIAN_POINT('Ctrl Pts',(1.48661551803772,0.0263496923375517,
132.338445777738));
#44347=CARTESIAN_POINT('Ctrl Pts',(1.49085937429597,-0.21310292201447,132.329470543168));
#44348=CARTESIAN_POINT('Ctrl Pts',(1.43607727001874,-0.453602335863666,
132.320495308598));
#44349=CARTESIAN_POINT('Ctrl Pts',(1.32854565172172,-0.667594747419045,
132.311520074027));
#44350=CARTESIAN_POINT('Ctrl Pts',(1.2210140334247,-0.881587158974429,132.302544839457));
#44351=CARTESIAN_POINT('Ctrl Pts',(1.06073290110789,-1.069072568236,132.293569604887));
#44352=CARTESIAN_POINT('Ctrl Pts',(0.866064757738101,-1.20857186741508,
132.284594370317));
#44353=CARTESIAN_POINT('Ctrl Pts',(0.671396614368315,-1.34807116659416,
132.275619135747));
#44354=CARTESIAN_POINT('Ctrl Pts',(0.442341459945558,-1.43958435569076,
132.266643901177));
#44355=CARTESIAN_POINT('Ctrl Pts',(0.20514125304273,-1.47262698657398,132.257668666607));
#44356=CARTESIAN_POINT('Ctrl Pts',(-0.0320589538600982,-1.5056696174572,
132.248693432037));
#44357=CARTESIAN_POINT('Ctrl Pts',(-0.277404213242995,-1.48024169012703,
132.239718197467));
#44358=CARTESIAN_POINT('Ctrl Pts',(-0.50278638102289,-1.399256442972,132.230742962896));
#44359=CARTESIAN_POINT('Ctrl Pts',(-0.728168548802785,-1.31827119581697,
132.221767728326));
#44360=CARTESIAN_POINT('Ctrl Pts',(-0.933587624979677,-1.18172862883706,
132.212792493756));
#44361=CARTESIAN_POINT('Ctrl Pts',(-1.09550958179572,-1.00527183024128,
132.203817259186));
#44362=CARTESIAN_POINT('Ctrl Pts',(-1.25743153861176,-0.828815031645493,
132.194842024616));
#44363=CARTESIAN_POINT('Ctrl Pts',(-1.37585637606696,-0.612444001433831,
132.185866790046));
#44364=CARTESIAN_POINT('Ctrl Pts',(-1.43721665915749,-0.38094749227848,
132.176891555476));
#44365=CARTESIAN_POINT('Ctrl Pts',(-1.47010769927003,-0.256858088106286,
132.172080547681));
#44366=CARTESIAN_POINT('Ctrl Pts',(-1.48660239861885,-0.128422684745344,
132.167269539885));
#44367=CARTESIAN_POINT('Ctrl Pts',(-1.48662495810528,7.0294833549589E-6,
132.16245853209));
#44368=CARTESIAN_POINT('Ctrl Pts',(-1.48667795283619,2.91850407830213E-5,
132.11254146791));
#44369=CARTESIAN_POINT('Ctrl Pts',(-1.48655244444886,-0.163132361450183,
132.118654163885));
#44370=CARTESIAN_POINT('Ctrl Pts',(-1.4597339032395,-0.326334184239694,
132.12476685986));
#44371=CARTESIAN_POINT('Ctrl Pts',(-1.40700263865445,-0.480683278165215,
132.130879555835));
#44372=CARTESIAN_POINT('Ctrl Pts',(-1.32957764144165,-0.707313120271662,
132.139854790405));
#44373=CARTESIAN_POINT('Ctrl Pts',(-1.19628773692095,-0.914857477991214,
132.148830024975));
#44374=CARTESIAN_POINT('Ctrl Pts',(-1.02240340176009,-1.07953884738407,
132.157805259545));
#44375=CARTESIAN_POINT('Ctrl Pts',(-0.848519066599234,-1.24422021677693,
132.166780494116));
#44376=CARTESIAN_POINT('Ctrl Pts',(-0.634040300798227,-1.3660385978431,
132.175755728686));
#44377=CARTESIAN_POINT('Ctrl Pts',(-0.403539054962874,-1.43103775907736,
132.184730963256));
#44378=CARTESIAN_POINT('Ctrl Pts',(-0.173037809127522,-1.49603692031162,
132.193706197826));
#44379=CARTESIAN_POINT('Ctrl Pts',(0.0734859167421764,-1.50421686171398,
132.202681432396));
#44380=CARTESIAN_POINT('Ctrl Pts',(0.307788911951766,-1.45464044142533,
132.211656666966));
#44381=CARTESIAN_POINT('Ctrl Pts',(0.542091907161356,-1.40506402113668,
132.220631901536));
#44382=CARTESIAN_POINT('Ctrl Pts',(0.764174171710838,-1.29773123915701,
132.229607136106));
#44383=CARTESIAN_POINT('Ctrl Pts',(0.948592653714135,-1.14493876981965,
132.238582370677));
#44384=CARTESIAN_POINT('Ctrl Pts',(1.13301113571743,-0.992146300482294,
132.247557605247));
#44385=CARTESIAN_POINT('Ctrl Pts',(1.27976583517455,-0.793894143787234,
132.256532839817));
#44386=CARTESIAN_POINT('Ctrl Pts',(1.37204366629816,-0.572895236586572,
132.265508074387));
#44387=CARTESIAN_POINT('Ctrl Pts',(1.46432149742177,-0.35189632938591,132.274483308957));
#44388=CARTESIAN_POINT('Ctrl Pts',(1.50212246021187,-0.108150671679646,
132.283458543527));
#44389=CARTESIAN_POINT('Ctrl Pts',(1.4811158560996,0.130416804746358,132.292433778097));
#44390=CARTESIAN_POINT('Ctrl Pts',(1.46010925198732,0.368984281172361,132.301409012667));
#44391=CARTESIAN_POINT('Ctrl Pts',(1.38029508097267,0.602373576318102,132.310384247238));
#44392=CARTESIAN_POINT('Ctrl Pts',(1.25081731064699,0.803846227062567,132.319359481808));
#44393=CARTESIAN_POINT('Ctrl Pts',(1.12133954032132,1.00531887780703,132.328334716378));
#44394=CARTESIAN_POINT('Ctrl Pts',(0.942198170684623,1.17487488415022,132.337309950948));
#44395=CARTESIAN_POINT('Ctrl Pts',(0.733916706066377,1.29308894190268,132.346285185518));
#44396=CARTESIAN_POINT('Ctrl Pts',(0.525635241448134,1.41130299965514,132.355260420088));
#44397=CARTESIAN_POINT('Ctrl Pts',(0.288213681848343,1.47817510881686,132.364235654658));
#44398=CARTESIAN_POINT('Ctrl Pts',(0.0488523752928705,1.48604395157025,
132.373210889228));
#44399=CARTESIAN_POINT('Ctrl Pts',(-0.190508931262602,1.49391279432363,
132.382186123798));
#44400=CARTESIAN_POINT('Ctrl Pts',(-0.431809984773757,1.44277837066867,
132.391161358369));
#44401=CARTESIAN_POINT('Ctrl Pts',(-0.647405838147634,1.33849908854363,
132.400136592939));
#44402=CARTESIAN_POINT('Ctrl Pts',(-0.863001691521512,1.23421980641859,
132.409111827509));
#44403=CARTESIAN_POINT('Ctrl Pts',(-1.05289234475811,1.07679566582346,132.418087062079));
#44404=CARTESIAN_POINT('Ctrl Pts',(-1.19532310554678,0.884261825513106,
132.427062296649));
#44405=CARTESIAN_POINT('Ctrl Pts',(-1.33775386633544,0.691727985202751,
132.436037531219));
#44406=CARTESIAN_POINT('Ctrl Pts',(-1.43272473467618,0.46408444517717,132.445012765789));
#44407=CARTESIAN_POINT('Ctrl Pts',(-1.46935487513581,0.227412102571081,
132.453988000359));
#44408=CARTESIAN_POINT('Ctrl Pts',(-1.48099114363096,0.152228581858804,
132.45683915621));
#44409=CARTESIAN_POINT('Ctrl Pts',(-1.48674003111915,0.0761339309162625,
132.45969031206));
#44410=CARTESIAN_POINT('Ctrl Pts',(-1.48668131839924,3.04819389219259E-5,
132.46254146791));
#44411=CARTESIAN_POINT('Origin',(0.,0.,130.353000754712));
#44412=CARTESIAN_POINT('',(-1.28651342453934,6.08325872239859E-6,132.278000754712));
#44413=CARTESIAN_POINT('',(-1.28656219828984,2.63788275486898E-5,132.346999245288));
#44414=CARTESIAN_POINT('',(-1.2866,7.40115670650129E-15,130.353000754712));
#44415=CARTESIAN_POINT('',(0.855148668267089,0.961251009262055,132.5));
#44416=CARTESIAN_POINT('Ctrl Pts',(-1.28651342453934,6.08325872233223E-6,
132.278000754712));
#44417=CARTESIAN_POINT('Ctrl Pts',(-1.28649390173904,-0.11113597080406,
132.282811762507));
#44418=CARTESIAN_POINT('Ctrl Pts',(-1.24558977217514,-0.429634554413405,
132.296598004872));
#44419=CARTESIAN_POINT('Ctrl Pts',(-0.98568734749738,-0.904495711840062,
132.319359481808));
#44420=CARTESIAN_POINT('Ctrl Pts',(-0.452383239321647,-1.25898426892294,
132.346285185518));
#44421=CARTESIAN_POINT('Ctrl Pts',(0.184576273813673,-1.32499964763048,
132.373210889228));
#44422=CARTESIAN_POINT('Ctrl Pts',(0.779243804823753,-1.08741528786317,
132.400136592939));
#44423=CARTESIAN_POINT('Ctrl Pts',(1.19536185928334,-0.600670138176585,
132.427062296649));
#44424=CARTESIAN_POINT('Ctrl Pts',(1.33758585234813,0.0237087063139161,
132.453988000359));
#44425=CARTESIAN_POINT('Ctrl Pts',(1.18926763353383,0.582583816218694,132.478300568143));
#44426=CARTESIAN_POINT('Ctrl Pts',(0.964859291222552,0.863480253952869,
132.493637901357));
#44427=CARTESIAN_POINT('Ctrl Pts',(0.855148668267089,0.961251009262055,
132.5));
#44428=CARTESIAN_POINT('',(1.18756226708949,-0.495010526943903,132.5));
#44429=CARTESIAN_POINT('Origin',(0.,0.,132.5));
#44430=CARTESIAN_POINT('Ctrl Pts',(-1.28656219828984,2.63788275487037E-5,
132.346999245288));
#44431=CARTESIAN_POINT('Ctrl Pts',(-1.28645306307448,-0.141434727128406,
132.353123324008));
#44432=CARTESIAN_POINT('Ctrl Pts',(-1.22901431635415,-0.490302866316248,
132.368222637298));
#44433=CARTESIAN_POINT('Ctrl Pts',(-0.919323220327711,-0.971881421552252,
132.392297185159));
#44434=CARTESIAN_POINT('Ctrl Pts',(-0.362304579342239,-1.28779095308542,
132.419222888869));
#44435=CARTESIAN_POINT('Ctrl Pts',(0.277699363289323,-1.30864921194912,
132.446148592579));
#44436=CARTESIAN_POINT('Ctrl Pts',(0.85410155756253,-1.02958919072608,132.47307429629));
#44437=CARTESIAN_POINT('Ctrl Pts',(1.10780466901396,-0.686354162750902,
132.49102476543));
#44438=CARTESIAN_POINT('Ctrl Pts',(1.18756226708949,-0.495010526943894,
132.5));
#44439=CARTESIAN_POINT('Origin',(0.,0.,130.353000754712));
#44440=CARTESIAN_POINT('',(-1.28651331007142,5.8758598133296E-6,131.928000754712));
#44441=CARTESIAN_POINT('',(-1.28655928575833,2.52565028640017E-5,131.996999245288));
#44442=CARTESIAN_POINT('',(-1.2866,7.40115670650129E-15,130.353000754712));
#44443=CARTESIAN_POINT('Ctrl Pts',(-1.28651331007142,5.87585981328548E-6,
131.928000754712));
#44444=CARTESIAN_POINT('Ctrl Pts',(-1.28649451528088,-0.110873252970274,
131.932800379762));
#44445=CARTESIAN_POINT('Ctrl Pts',(-1.24572312673905,-0.429108439932022,
131.946575239382));
#44446=CARTESIAN_POINT('Ctrl Pts',(-0.986241701669955,-0.903891264481546,
131.969325333573));
#44447=CARTESIAN_POINT('Ctrl Pts',(-0.453155086833697,-1.25870670904991,
131.996251037283));
#44448=CARTESIAN_POINT('Ctrl Pts',(0.183763759504555,-1.32511244536446,
132.023176740994));
#44449=CARTESIAN_POINT('Ctrl Pts',(0.778576488622803,-1.08789280890088,
132.050102444704));
#44450=CARTESIAN_POINT('Ctrl Pts',(1.1949926014029,-0.601402357101034,132.077028148414));
#44451=CARTESIAN_POINT('Ctrl Pts',(1.3375979328864,0.02288848698503,132.103953852125));
#44452=CARTESIAN_POINT('Ctrl Pts',(1.17371706985718,0.641934851359759,132.130879555835));
#44453=CARTESIAN_POINT('Ctrl Pts',(0.740900326155663,1.11389354058136,132.157805259545));
#44454=CARTESIAN_POINT('Ctrl Pts',(0.138319773232647,1.3306238208134,132.184730963256));
#44455=CARTESIAN_POINT('Ctrl Pts',(-0.495954234429353,1.24246589576165,
132.211656666966));
#44456=CARTESIAN_POINT('Ctrl Pts',(-1.01658936156519,0.869619550362351,
132.238582370677));
#44457=CARTESIAN_POINT('Ctrl Pts',(-1.25288574974687,0.399737600901963,
132.260697066592));
#44458=CARTESIAN_POINT('Ctrl Pts',(-1.28653032273847,0.0962064506343579,
132.273836527937));
#44459=CARTESIAN_POINT('Ctrl Pts',(-1.28651342453934,6.08325872233223E-6,
132.278000754712));
#44460=CARTESIAN_POINT('Ctrl Pts',(-1.28655928575833,2.52565028640434E-5,
131.996999245288));
#44461=CARTESIAN_POINT('Ctrl Pts',(-1.28645067179739,-0.14117344918617,
132.003111941263));
#44462=CARTESIAN_POINT('Ctrl Pts',(-1.22916514203553,-0.489779393246562,
132.018199871809));
#44463=CARTESIAN_POINT('Ctrl Pts',(-0.919909876517952,-0.971317628899406,
132.042263036924));
#44464=CARTESIAN_POINT('Ctrl Pts',(-0.363085218132085,-1.28757960555225,
132.069188740634));
#44465=CARTESIAN_POINT('Ctrl Pts',(0.276933801600455,-1.30881617440312,
132.096114444345));
#44466=CARTESIAN_POINT('Ctrl Pts',(0.853498482162152,-1.0301613647476,132.123040148055));
#44467=CARTESIAN_POINT('Ctrl Pts',(1.23449953411498,-0.51546384206413,132.149965851765));
#44468=CARTESIAN_POINT('Ctrl Pts',(1.33263749249817,0.117342823334407,132.176891555476));
#44469=CARTESIAN_POINT('Ctrl Pts',(1.125425844559,0.72326254715928,132.203817259186));
#44470=CARTESIAN_POINT('Ctrl Pts',(0.660343291616316,1.16345980844394,132.230742962896));
#44471=CARTESIAN_POINT('Ctrl Pts',(0.0439550989490249,1.33707158395214,
132.257668666607));
#44472=CARTESIAN_POINT('Ctrl Pts',(-0.582504943319958,1.20431761235457,
132.284594370317));
#44473=CARTESIAN_POINT('Ctrl Pts',(-1.07549453007113,0.795616811689296,
132.311520074027));
#44474=CARTESIAN_POINT('Ctrl Pts',(-1.2659768915234,0.339033863349242,132.332321699018));
#44475=CARTESIAN_POINT('Ctrl Pts',(-1.28661300781106,0.065885698778665,
132.344148089438));
#44476=CARTESIAN_POINT('Ctrl Pts',(-1.28656219828984,2.63788275487037E-5,
132.346999245288));
#44477=CARTESIAN_POINT('Origin',(0.,0.,130.353000754712));
#44478=CARTESIAN_POINT('',(-1.28651317526843,5.66436777652892E-6,131.578000754712));
#44479=CARTESIAN_POINT('',(-1.28655866463832,2.51533884142174E-5,131.646999245288));
#44480=CARTESIAN_POINT('',(-1.2866,7.40115670650129E-15,130.353000754712));
#44481=CARTESIAN_POINT('Ctrl Pts',(-1.28651317526843,5.66436777649226E-6,
131.578000754712));
#44482=CARTESIAN_POINT('Ctrl Pts',(-1.28649510270387,-0.110610537845435,
131.582788997017));
#44483=CARTESIAN_POINT('Ctrl Pts',(-1.24585626516315,-0.428582328169219,
131.596552473893));
#44484=CARTESIAN_POINT('Ctrl Pts',(-0.986795626701916,-0.903286501201301,
131.619291185338));
#44485=CARTESIAN_POINT('Ctrl Pts',(-0.453926623709776,-1.25842867593135,
131.646216889049));
#44486=CARTESIAN_POINT('Ctrl Pts',(0.182951394380693,-1.3252248486269,131.673142592759));
#44487=CARTESIAN_POINT('Ctrl Pts',(0.777909433892818,-1.08836989336796,
131.700068296469));
#44488=CARTESIAN_POINT('Ctrl Pts',(1.19462370043953,-0.602134807565142,
131.72699400018));
#44489=CARTESIAN_POINT('Ctrl Pts',(1.33761171253848,0.0220684982618089,
131.75391970389));
#44490=CARTESIAN_POINT('Ctrl Pts',(1.17411037251451,0.641215209809031,131.7808454076));
#44491=CARTESIAN_POINT('Ctrl Pts',(0.741583033376361,1.11343913921922,131.807771111311));
#44492=CARTESIAN_POINT('Ctrl Pts',(0.139135454071305,1.33053877717148,131.834696815021));
#44493=CARTESIAN_POINT('Ctrl Pts',(-0.495192479431881,1.24276969726887,
131.861622518732));
#44494=CARTESIAN_POINT('Ctrl Pts',(-1.01605607887236,0.870242584984128,
131.888548222442));
#44495=CARTESIAN_POINT('Ctrl Pts',(-1.25276225187591,0.400263803823439,
131.910674301102));
#44496=CARTESIAN_POINT('Ctrl Pts',(-1.28652966128751,0.0964692331083593,
131.923825145192));
#44497=CARTESIAN_POINT('Ctrl Pts',(-1.28651331007142,5.87585981328548E-6,
131.928000754712));
#44498=CARTESIAN_POINT('Ctrl Pts',(-1.28655866463832,2.51533884142105E-5,
131.646999245288));
#44499=CARTESIAN_POINT('Ctrl Pts',(-1.28645078202246,-0.140910814969984,
131.653100558519));
#44500=CARTESIAN_POINT('Ctrl Pts',(-1.22931900951945,-0.489253663809912,
131.668177106319));
#44501=CARTESIAN_POINT('Ctrl Pts',(-0.920505147196365,-0.970753516707333,
131.692228888689));
#44502=CARTESIAN_POINT('Ctrl Pts',(-0.363874469513489,-1.2873567829668,
131.7191545924));
#44503=CARTESIAN_POINT('Ctrl Pts',(0.276131412923829,-1.30898569855063,
131.74608029611));
#44504=CARTESIAN_POINT('Ctrl Pts',(0.852866813310974,-1.03068439153984,
131.77300599982));
#44505=CARTESIAN_POINT('Ctrl Pts',(1.23418332299191,-0.516220535677922,
131.799931703531));
#44506=CARTESIAN_POINT('Ctrl Pts',(1.33270921150778,0.116525850196642,131.826857407241));
#44507=CARTESIAN_POINT('Ctrl Pts',(1.12586906668276,0.722572460645641,131.853783110951));
#44508=CARTESIAN_POINT('Ctrl Pts',(0.661056538993872,1.16305475729291,131.880708814662));
#44509=CARTESIAN_POINT('Ctrl Pts',(0.0447749500858785,1.33704424761847,
131.907634518372));
#44510=CARTESIAN_POINT('Ctrl Pts',(-0.581766002838075,1.20467441008527,
131.934560222082));
#44511=CARTESIAN_POINT('Ctrl Pts',(-1.07500587627816,0.796275381121529,
131.961485925793));
#44512=CARTESIAN_POINT('Ctrl Pts',(-1.26587133036338,0.339559855102084,
131.982298933528));
#44513=CARTESIAN_POINT('Ctrl Pts',(-1.28661014902004,0.0661477573208332,
131.994136706693));
#44514=CARTESIAN_POINT('Ctrl Pts',(-1.28655928575833,2.52565028640434E-5,
131.996999245288));
#44515=CARTESIAN_POINT('Origin',(0.,0.,130.353000754712));
#44516=CARTESIAN_POINT('',(-1.28651324097226,5.80358258384201E-6,131.228000754712));
#44517=CARTESIAN_POINT('',(-1.28655804524971,2.50455016348461E-5,131.296999245288));
#44518=CARTESIAN_POINT('',(-1.2866,7.40115670650129E-15,130.353000754712));
#44519=CARTESIAN_POINT('Ctrl Pts',(-1.28651324097226,5.80358258382013E-6,
131.228000754712));
#44520=CARTESIAN_POINT('Ctrl Pts',(-1.28649587088415,-0.110347520289303,
131.232777614272));
#44521=CARTESIAN_POINT('Ctrl Pts',(-1.24598938676408,-0.428056057830857,
131.246529708403));
#44522=CARTESIAN_POINT('Ctrl Pts',(-0.98734923478118,-0.902681268882645,
131.269257037104));
#44523=CARTESIAN_POINT('Ctrl Pts',(-0.454698034476922,-1.2581501250631,
131.296182740814));
#44524=CARTESIAN_POINT('Ctrl Pts',(0.182138945505527,-1.32533672141841,
131.323108444524));
#44525=CARTESIAN_POINT('Ctrl Pts',(0.777242075774215,-1.08884655660415,
131.350034148235));
#44526=CARTESIAN_POINT('Ctrl Pts',(1.19425434657027,-0.602867023578126,
131.376959851945));
#44527=CARTESIAN_POINT('Ctrl Pts',(1.33762498699637,0.0212485044686996,
131.403885555655));
#44528=CARTESIAN_POINT('Ctrl Pts',(1.17450323342847,0.640495329295421,131.430811259366));
#44529=CARTESIAN_POINT('Ctrl Pts',(0.742265462285602,1.11298431999035,131.457736963076));
#44530=CARTESIAN_POINT('Ctrl Pts',(0.139951084671291,1.3304532338131,131.484662666786));
#44531=CARTESIAN_POINT('Ctrl Pts',(-0.494430534395506,1.24307303066064,
131.511588370497));
#44532=CARTESIAN_POINT('Ctrl Pts',(-1.01552240527922,0.870865292057418,
131.538514074207));
#44533=CARTESIAN_POINT('Ctrl Pts',(-1.25263856527262,0.400790001029229,
131.560651535612));
#44534=CARTESIAN_POINT('Ctrl Pts',(-1.28652897849709,0.0967320105866091,
131.573813762447));
#44535=CARTESIAN_POINT('Ctrl Pts',(-1.28651317526843,5.66436777649226E-6,
131.578000754712));
#44536=CARTESIAN_POINT('Ctrl Pts',(-1.28655804524971,2.50455016348322E-5,
131.296999245288));
#44537=CARTESIAN_POINT('Ctrl Pts',(-1.28645089716158,-0.14064818329876,
131.303089175774));
#44538=CARTESIAN_POINT('Ctrl Pts',(-1.22947269431557,-0.488727931596862,
131.318154340829));
#44539=CARTESIAN_POINT('Ctrl Pts',(-0.92110007241593,-0.970189040198561,
131.342194740455));
#44540=CARTESIAN_POINT('Ctrl Pts',(-0.364663586223146,-1.28713347653886,
131.369120444165));
#44541=CARTESIAN_POINT('Ctrl Pts',(0.275328916768196,-1.30915472904038,
131.396046147875));
#44542=CARTESIAN_POINT('Ctrl Pts',(0.852234815095578,-1.03120702894802,
131.422971851586));
#44543=CARTESIAN_POINT('Ctrl Pts',(1.23386663366973,-0.516977027235267,
131.449897555296));
#44544=CARTESIAN_POINT('Ctrl Pts',(1.332780394676,0.115708840682625,131.476823259006));
#44545=CARTESIAN_POINT('Ctrl Pts',(1.1263118120373,0.721882135998308,131.503748962717));
#44546=CARTESIAN_POINT('Ctrl Pts',(0.661769399512303,1.16264929280748,131.530674666427));
#44547=CARTESIAN_POINT('Ctrl Pts',(0.0455945867891589,1.33701654808655,
131.557600370137));
#44548=CARTESIAN_POINT('Ctrl Pts',(-0.581027394744716,1.20503082232908,
131.584526073848));
#44549=CARTESIAN_POINT('Ctrl Pts',(-1.07451753531689,0.796934239763604,
131.611451777558));
#44550=CARTESIAN_POINT('Ctrl Pts',(-1.26576747112306,0.340086089182502,
131.632276168038));
#44551=CARTESIAN_POINT('Ctrl Pts',(-1.28660948093643,0.0664106792179535,
131.644125323948));
#44552=CARTESIAN_POINT('Ctrl Pts',(-1.28655866463832,2.51533884142105E-5,
131.646999245288));
#44553=CARTESIAN_POINT('Origin',(1.88724897194442,-1.29707028255787,134.));
#44554=CARTESIAN_POINT('',(1.8802655232717,-1.2357595081551,132.6));
#44555=CARTESIAN_POINT('',(1.8802655232717,-1.23575950815512,133.85));
#44556=CARTESIAN_POINT('',(1.8802655232717,-1.23575950815512,133.225));
#44557=CARTESIAN_POINT('',(1.86195461813654,-1.075,132.6));
#44558=CARTESIAN_POINT('',(1.88724897194442,-1.29707028255787,132.6));
#44559=CARTESIAN_POINT('',(1.86195461813654,-1.075,133.95));
#44560=CARTESIAN_POINT('',(1.86195461813654,-1.075,134.));
#44561=CARTESIAN_POINT('Ctrl Pts',(1.8802655232717,-1.23575950815514,133.85));
#44562=CARTESIAN_POINT('Ctrl Pts',(1.87090199223673,-1.15355294148538,133.902974875989));
#44563=CARTESIAN_POINT('Ctrl Pts',(1.86195461813654,-1.075,133.95));
#44564=CARTESIAN_POINT('Origin',(1.86195461813654,-1.075,134.));
#44565=CARTESIAN_POINT('',(2.01033188866635,-1.01047795493577,133.85));
#44566=CARTESIAN_POINT('Ctrl Pts',(1.86195461813654,-1.075,133.95));
#44567=CARTESIAN_POINT('Ctrl Pts',(1.93445714805536,-1.04347218252507,133.902974875989));
#44568=CARTESIAN_POINT('Ctrl Pts',(2.01033188866637,-1.01047795493577,133.85));
#44569=CARTESIAN_POINT('',(2.01033188866633,-1.01047795493578,132.6));
#44570=CARTESIAN_POINT('',(1.86195461813654,-1.075,132.6));
#44571=CARTESIAN_POINT('',(2.01033188866635,-1.01047795493577,133.225));
#44572=CARTESIAN_POINT('Origin',(1.96443745964886,-1.14147034712443,132.6));
#44573=CARTESIAN_POINT('Origin',(0.,0.,132.6));
#44574=CARTESIAN_POINT('Origin',(0.985870411690995,-2.06692030116118,134.));
#44575=CARTESIAN_POINT('',(1.01047795493578,-2.01033188866633,132.6));
#44576=CARTESIAN_POINT('',(1.01047795493577,-2.01033188866635,133.85));
#44577=CARTESIAN_POINT('',(1.01047795493577,-2.01033188866635,133.225));
#44578=CARTESIAN_POINT('',(1.075,-1.86195461813654,132.6));
#44579=CARTESIAN_POINT('',(0.985870411690995,-2.06692030116118,132.6));
#44580=CARTESIAN_POINT('',(1.075,-1.86195461813654,133.95));
#44581=CARTESIAN_POINT('',(1.075,-1.86195461813654,134.));
#44582=CARTESIAN_POINT('Ctrl Pts',(1.01047795493577,-2.01033188866637,133.85));
#44583=CARTESIAN_POINT('Ctrl Pts',(1.04347218252507,-1.93445714805537,133.902974875989));
#44584=CARTESIAN_POINT('Ctrl Pts',(1.075,-1.86195461813654,133.95));
#44585=CARTESIAN_POINT('Origin',(1.075,-1.86195461813654,134.));
#44586=CARTESIAN_POINT('',(1.23575950815512,-1.8802655232717,133.85));
#44587=CARTESIAN_POINT('Ctrl Pts',(1.075,-1.86195461813654,133.95));
#44588=CARTESIAN_POINT('Ctrl Pts',(1.1535529414858,-1.87090199223678,133.902974875989));
#44589=CARTESIAN_POINT('Ctrl Pts',(1.23575950815514,-1.88026552327171,133.85));
#44590=CARTESIAN_POINT('',(1.2357595081551,-1.8802655232717,132.6));
#44591=CARTESIAN_POINT('',(1.075,-1.86195461813654,132.6));
#44592=CARTESIAN_POINT('',(1.23575950815512,-1.8802655232717,133.225));
#44593=CARTESIAN_POINT('Origin',(1.14147034712443,-1.96443745964886,132.6));
#44594=CARTESIAN_POINT('Origin',(0.,0.,132.6));
#44595=CARTESIAN_POINT('Origin',(-0.179671329216764,-2.28294069424886,134.));
#44596=CARTESIAN_POINT('',(-0.13006636539463,-2.24623746309088,132.6));
#44597=CARTESIAN_POINT('',(-0.130066365394647,-2.2462374630909,133.85));
#44598=CARTESIAN_POINT('',(-0.130066365394647,-2.2462374630909,133.225));
#44599=CARTESIAN_POINT('',(-3.94948592725021E-16,-2.15,132.6));
#44600=CARTESIAN_POINT('',(-0.179671329216764,-2.28294069424886,132.6));
#44601=CARTESIAN_POINT('',(-3.94948592725021E-16,-2.15,133.95));
#44602=CARTESIAN_POINT('',(-3.94948592725021E-16,-2.15,134.));
#44603=CARTESIAN_POINT('Ctrl Pts',(-0.130066365394665,-2.24623746309091,
133.85));
#44604=CARTESIAN_POINT('Ctrl Pts',(-0.0635551558182033,-2.19702512401059,
133.902974875989));
#44605=CARTESIAN_POINT('Ctrl Pts',(-3.94948592725021E-16,-2.15,133.95));
#44606=CARTESIAN_POINT('Origin',(-3.94948592725021E-16,-2.15,134.));
#44607=CARTESIAN_POINT('',(0.130066365394648,-2.2462374630909,133.85));
#44608=CARTESIAN_POINT('Ctrl Pts',(-3.94948592725021E-16,-2.15,133.95));
#44609=CARTESIAN_POINT('Ctrl Pts',(0.0635551558186,-2.19702512401089,133.902974875989));
#44610=CARTESIAN_POINT('Ctrl Pts',(0.130066365394665,-2.24623746309091,
133.85));
#44611=CARTESIAN_POINT('',(0.13006636539463,-2.24623746309088,132.6));
#44612=CARTESIAN_POINT('',(-3.94948592725021E-16,-2.15,132.6));
#44613=CARTESIAN_POINT('',(0.130066365394648,-2.2462374630909,133.225));
#44614=CARTESIAN_POINT('Origin',(6.10622663543836E-16,-2.21647034712443,
132.6));
#44615=CARTESIAN_POINT('Origin',(0.,0.,132.6));
#44616=CARTESIAN_POINT('Origin',(-1.29707028255787,-1.88724897194442,134.));
#44617=CARTESIAN_POINT('',(-1.2357595081551,-1.8802655232717,132.6));
#44618=CARTESIAN_POINT('',(-1.23575950815512,-1.8802655232717,133.85));
#44619=CARTESIAN_POINT('',(-1.23575950815512,-1.8802655232717,133.225));
#44620=CARTESIAN_POINT('',(-1.075,-1.86195461813654,132.6));
#44621=CARTESIAN_POINT('',(-1.29707028255787,-1.88724897194442,132.6));
#44622=CARTESIAN_POINT('',(-1.075,-1.86195461813654,133.95));
#44623=CARTESIAN_POINT('',(-1.075,-1.86195461813654,134.));
#44624=CARTESIAN_POINT('Ctrl Pts',(-1.23575950815514,-1.8802655232717,133.85));
#44625=CARTESIAN_POINT('Ctrl Pts',(-1.15355294148538,-1.87090199223673,
133.902974875989));
#44626=CARTESIAN_POINT('Ctrl Pts',(-1.075,-1.86195461813654,133.95));
#44627=CARTESIAN_POINT('Origin',(-1.075,-1.86195461813654,134.));
#44628=CARTESIAN_POINT('',(-1.01047795493577,-2.01033188866635,133.85));
#44629=CARTESIAN_POINT('Ctrl Pts',(-1.075,-1.86195461813654,133.95));
#44630=CARTESIAN_POINT('Ctrl Pts',(-1.04347218252507,-1.93445714805536,
133.902974875989));
#44631=CARTESIAN_POINT('Ctrl Pts',(-1.01047795493577,-2.01033188866637,
133.85));
#44632=CARTESIAN_POINT('',(-1.01047795493578,-2.01033188866633,132.6));
#44633=CARTESIAN_POINT('',(-1.075,-1.86195461813654,132.6));
#44634=CARTESIAN_POINT('',(-1.01047795493577,-2.01033188866635,133.225));
#44635=CARTESIAN_POINT('Origin',(-1.14147034712443,-1.96443745964886,132.6));
#44636=CARTESIAN_POINT('Origin',(0.,0.,132.6));
#44637=CARTESIAN_POINT('Origin',(-2.06692030116118,-0.985870411690996,134.));
#44638=CARTESIAN_POINT('',(-2.01033188866633,-1.01047795493578,132.6));
#44639=CARTESIAN_POINT('',(-2.01033188866635,-1.01047795493577,133.85));
#44640=CARTESIAN_POINT('',(-2.01033188866635,-1.01047795493577,133.225));
#44641=CARTESIAN_POINT('',(-1.86195461813654,-1.075,132.6));
#44642=CARTESIAN_POINT('',(-2.06692030116118,-0.985870411690996,132.6));
#44643=CARTESIAN_POINT('',(-1.86195461813654,-1.075,133.95));
#44644=CARTESIAN_POINT('',(-1.86195461813654,-1.075,134.));
#44645=CARTESIAN_POINT('Ctrl Pts',(-2.01033188866637,-1.01047795493577,
133.85));
#44646=CARTESIAN_POINT('Ctrl Pts',(-1.93445714805536,-1.04347218252507,
133.902974875989));
#44647=CARTESIAN_POINT('Ctrl Pts',(-1.86195461813654,-1.075,133.95));
#44648=CARTESIAN_POINT('Origin',(-1.86195461813654,-1.075,134.));
#44649=CARTESIAN_POINT('',(-1.8802655232717,-1.23575950815512,133.85));
#44650=CARTESIAN_POINT('Ctrl Pts',(-1.86195461813654,-1.075,133.95));
#44651=CARTESIAN_POINT('Ctrl Pts',(-1.87090199223678,-1.15355294148581,
133.902974875989));
#44652=CARTESIAN_POINT('Ctrl Pts',(-1.88026552327171,-1.23575950815514,
133.85));
#44653=CARTESIAN_POINT('',(-1.8802655232717,-1.2357595081551,132.6));
#44654=CARTESIAN_POINT('',(-1.86195461813654,-1.075,132.6));
#44655=CARTESIAN_POINT('',(-1.8802655232717,-1.23575950815512,133.225));
#44656=CARTESIAN_POINT('Origin',(-1.96443745964886,-1.14147034712443,132.6));
#44657=CARTESIAN_POINT('Origin',(0.,0.,132.6));
#44658=CARTESIAN_POINT('Origin',(-2.28294069424886,0.179671329216765,134.));
#44659=CARTESIAN_POINT('',(-2.24623746309088,0.13006636539463,132.6));
#44660=CARTESIAN_POINT('',(-2.2462374630909,0.130066365394648,133.85));
#44661=CARTESIAN_POINT('',(-2.2462374630909,0.130066365394648,133.225));
#44662=CARTESIAN_POINT('',(-2.15,2.63299061816681E-16,132.6));
#44663=CARTESIAN_POINT('',(-2.28294069424886,0.179671329216765,132.6));
#44664=CARTESIAN_POINT('',(-2.15,2.63299061816681E-16,133.95));
#44665=CARTESIAN_POINT('',(-2.15,2.63299061816681E-16,134.));
#44666=CARTESIAN_POINT('Ctrl Pts',(-2.24623746309091,0.130066365394665,
133.85));
#44667=CARTESIAN_POINT('Ctrl Pts',(-2.19702512401088,0.0635551558185912,
133.902974875989));
#44668=CARTESIAN_POINT('Ctrl Pts',(-2.15,2.63299061816681E-16,133.95));
#44669=CARTESIAN_POINT('Origin',(-2.15,2.63299061816681E-16,134.));
#44670=CARTESIAN_POINT('',(-2.2462374630909,-0.130066365394647,133.85));
#44671=CARTESIAN_POINT('Ctrl Pts',(-2.15,2.63299061816681E-16,133.95));
#44672=CARTESIAN_POINT('Ctrl Pts',(-2.19702512401089,-0.0635551558186091,
133.902974875989));
#44673=CARTESIAN_POINT('Ctrl Pts',(-2.24623746309091,-0.130066365394664,
133.85));
#44674=CARTESIAN_POINT('',(-2.24623746309088,-0.13006636539463,132.6));
#44675=CARTESIAN_POINT('',(-2.15,2.63299061816681E-16,132.6));
#44676=CARTESIAN_POINT('',(-2.2462374630909,-0.130066365394647,133.225));
#44677=CARTESIAN_POINT('Origin',(-2.21647034712443,2.77555756156289E-16,
132.6));
#44678=CARTESIAN_POINT('',(-2.24999999999999,-2.75545529808154E-16,132.6));
#44679=CARTESIAN_POINT('Origin',(0.,0.,132.6));
#44680=CARTESIAN_POINT('Origin',(0.,0.,132.6));
#44681=CARTESIAN_POINT('Origin',(-2.15864901460109,0.764417707645336,134.));
#44682=CARTESIAN_POINT('',(-2.13603512508613,0.707003496736915,132.6));
#44683=CARTESIAN_POINT('',(-2.13603512508614,0.707003496736936,133.85));
#44684=CARTESIAN_POINT('',(-2.13603512508614,0.707003496736936,133.225));
#44685=CARTESIAN_POINT('',(-2.0767405265215,0.55646094697042,132.6));
#44686=CARTESIAN_POINT('',(-2.15864901460109,0.764417707645336,132.6));
#44687=CARTESIAN_POINT('',(-2.0767405265215,0.55646094697042,133.95));
#44688=CARTESIAN_POINT('',(-2.0767405265215,0.55646094697042,134.));
#44689=CARTESIAN_POINT('Ctrl Pts',(-2.13603512508614,0.707003496736955,
133.85));
#44690=CARTESIAN_POINT('Ctrl Pts',(-2.10571402354774,0.63002151106175,133.902974875989));
#44691=CARTESIAN_POINT('Ctrl Pts',(-2.0767405265215,0.55646094697042,133.95));
#44692=CARTESIAN_POINT('Origin',(-2.0767405265215,0.55646094697042,134.));
#44693=CARTESIAN_POINT('',(-2.20336243006893,0.455734573804454,133.85));
#44694=CARTESIAN_POINT('Ctrl Pts',(-2.0767405265215,0.55646094697042,133.95));
#44695=CARTESIAN_POINT('Ctrl Pts',(-2.13861259302839,0.50724237826372,133.902974875989));
#44696=CARTESIAN_POINT('Ctrl Pts',(-2.20336243006895,0.455734573804441,
133.85));
#44697=CARTESIAN_POINT('',(-2.20336243006892,0.455734573804468,132.6));
#44698=CARTESIAN_POINT('',(-2.0767405265215,0.55646094697042,132.6));
#44699=CARTESIAN_POINT('',(-2.20336243006893,0.455734573804454,133.225));
#44700=CARTESIAN_POINT('Origin',(-2.16419713242148,0.590868530511177,132.6));
#44701=CARTESIAN_POINT('Origin',(0.,0.,132.6));
#44702=CARTESIAN_POINT('Origin',(-1.48723603067612,1.74132966122407,134.));
#44703=CARTESIAN_POINT('',(-1.496358933332,1.68030055128166,132.6));
#44704=CARTESIAN_POINT('',(-1.496358933332,1.68030055128168,133.85));
#44705=CARTESIAN_POINT('',(-1.496358933332,1.68030055128168,133.225));
#44706=CARTESIAN_POINT('',(-1.52027957955108,1.52027957955108,132.6));
#44707=CARTESIAN_POINT('',(-1.48723603067612,1.74132966122407,132.6));
#44708=CARTESIAN_POINT('',(-1.52027957955108,1.52027957955108,133.95));
#44709=CARTESIAN_POINT('',(-1.52027957955108,1.52027957955108,134.));
#44710=CARTESIAN_POINT('Ctrl Pts',(-1.49635893333199,1.6803005512817,133.85));
#44711=CARTESIAN_POINT('Ctrl Pts',(-1.50859108196662,1.598471645284,133.902974875989));
#44712=CARTESIAN_POINT('Ctrl Pts',(-1.52027957955108,1.52027957955108,133.95));
#44713=CARTESIAN_POINT('Origin',(-1.52027957955108,1.52027957955108,134.));
#44714=CARTESIAN_POINT('',(-1.68030055128168,1.496358933332,133.85));
#44715=CARTESIAN_POINT('Ctrl Pts',(-1.52027957955108,1.52027957955108,133.95));
#44716=CARTESIAN_POINT('Ctrl Pts',(-1.59847164528371,1.50859108196666,133.902974875989));
#44717=CARTESIAN_POINT('Ctrl Pts',(-1.6803005512817,1.49635893333199,133.85));
#44718=CARTESIAN_POINT('',(-1.68030055128166,1.496358933332,132.6));
#44719=CARTESIAN_POINT('',(-1.52027957955108,1.52027957955108,132.6));
#44720=CARTESIAN_POINT('',(-1.68030055128168,1.496358933332,133.225));
#44721=CARTESIAN_POINT('Origin',(-1.6142828459501,1.6142828459501,132.6));
#44722=CARTESIAN_POINT('Origin',(0.,0.,132.6));
#44723=CARTESIAN_POINT('Origin',(-0.417319353377018,2.25165373832146,134.));
#44724=CARTESIAN_POINT('',(-0.455734573804468,2.20336243006892,132.6));
#44725=CARTESIAN_POINT('',(-0.455734573804454,2.20336243006893,133.85));
#44726=CARTESIAN_POINT('',(-0.455734573804454,2.20336243006893,133.225));
#44727=CARTESIAN_POINT('',(-0.55646094697042,2.0767405265215,132.6));
#44728=CARTESIAN_POINT('',(-0.417319353377018,2.25165373832146,132.6));
#44729=CARTESIAN_POINT('',(-0.55646094697042,2.0767405265215,133.95));
#44730=CARTESIAN_POINT('',(-0.55646094697042,2.0767405265215,134.));
#44731=CARTESIAN_POINT('Ctrl Pts',(-0.455734573804441,2.20336243006895,
133.85));
#44732=CARTESIAN_POINT('Ctrl Pts',(-0.507242378263725,2.13861259302838,
133.902974875989));
#44733=CARTESIAN_POINT('Ctrl Pts',(-0.55646094697042,2.0767405265215,133.95));
#44734=CARTESIAN_POINT('Origin',(-0.55646094697042,2.0767405265215,134.));
#44735=CARTESIAN_POINT('',(-0.707003496736936,2.13603512508614,133.85));
#44736=CARTESIAN_POINT('Ctrl Pts',(-0.55646094697042,2.0767405265215,133.95));
#44737=CARTESIAN_POINT('Ctrl Pts',(-0.630021511061762,2.10571402354775,
133.902974875989));
#44738=CARTESIAN_POINT('Ctrl Pts',(-0.707003496736956,2.13603512508614,
133.85));
#44739=CARTESIAN_POINT('',(-0.707003496736916,2.13603512508613,132.6));
#44740=CARTESIAN_POINT('',(-0.55646094697042,2.0767405265215,132.6));
#44741=CARTESIAN_POINT('',(-0.707003496736936,2.13603512508614,133.225));
#44742=CARTESIAN_POINT('Origin',(-0.590868530511177,2.16419713242148,132.6));
#44743=CARTESIAN_POINT('Origin',(0.,0.,132.6));
#44744=CARTESIAN_POINT('Origin',(0.764417707645335,2.15864901460109,134.));
#44745=CARTESIAN_POINT('',(0.707003496736915,2.13603512508613,132.6));
#44746=CARTESIAN_POINT('',(0.707003496736935,2.13603512508614,133.85));
#44747=CARTESIAN_POINT('',(0.707003496736935,2.13603512508614,133.225));
#44748=CARTESIAN_POINT('',(0.55646094697042,2.0767405265215,132.6));
#44749=CARTESIAN_POINT('',(0.764417707645335,2.15864901460109,132.6));
#44750=CARTESIAN_POINT('',(0.55646094697042,2.0767405265215,133.95));
#44751=CARTESIAN_POINT('',(0.55646094697042,2.0767405265215,134.));
#44752=CARTESIAN_POINT('Ctrl Pts',(0.707003496736955,2.13603512508614,133.85));
#44753=CARTESIAN_POINT('Ctrl Pts',(0.630021511061745,2.10571402354774,133.902974875989));
#44754=CARTESIAN_POINT('Ctrl Pts',(0.55646094697042,2.0767405265215,133.95));
#44755=CARTESIAN_POINT('Origin',(0.55646094697042,2.0767405265215,134.));
#44756=CARTESIAN_POINT('',(0.455734573804454,2.20336243006893,133.85));
#44757=CARTESIAN_POINT('Ctrl Pts',(0.55646094697042,2.0767405265215,133.95));
#44758=CARTESIAN_POINT('Ctrl Pts',(0.507242378263745,2.13861259302836,133.902974875989));
#44759=CARTESIAN_POINT('Ctrl Pts',(0.45573457380444,2.20336243006895,133.85));
#44760=CARTESIAN_POINT('',(0.455734573804467,2.20336243006892,132.6));
#44761=CARTESIAN_POINT('',(0.55646094697042,2.0767405265215,132.6));
#44762=CARTESIAN_POINT('',(0.455734573804454,2.20336243006893,133.225));
#44763=CARTESIAN_POINT('Origin',(0.590868530511176,2.16419713242148,132.6));
#44764=CARTESIAN_POINT('Origin',(0.,0.,132.6));
#44765=CARTESIAN_POINT('Origin',(1.74132966122407,1.48723603067612,134.));
#44766=CARTESIAN_POINT('',(1.68030055128166,1.496358933332,132.6));
#44767=CARTESIAN_POINT('',(1.68030055128168,1.496358933332,133.85));
#44768=CARTESIAN_POINT('',(1.68030055128168,1.496358933332,133.225));
#44769=CARTESIAN_POINT('',(1.52027957955108,1.52027957955108,132.6));
#44770=CARTESIAN_POINT('',(1.74132966122407,1.48723603067612,132.6));
#44771=CARTESIAN_POINT('',(1.52027957955108,1.52027957955108,133.95));
#44772=CARTESIAN_POINT('',(1.52027957955108,1.52027957955108,134.));
#44773=CARTESIAN_POINT('Ctrl Pts',(1.6803005512817,1.49635893333199,133.85));
#44774=CARTESIAN_POINT('Ctrl Pts',(1.59847164528401,1.50859108196661,133.902974875989));
#44775=CARTESIAN_POINT('Ctrl Pts',(1.52027957955108,1.52027957955108,133.95));
#44776=CARTESIAN_POINT('Origin',(1.52027957955108,1.52027957955108,134.));
#44777=CARTESIAN_POINT('',(1.496358933332,1.68030055128168,133.85));
#44778=CARTESIAN_POINT('Ctrl Pts',(1.52027957955108,1.52027957955108,133.95));
#44779=CARTESIAN_POINT('Ctrl Pts',(1.50859108196669,1.59847164528354,133.902974875989));
#44780=CARTESIAN_POINT('Ctrl Pts',(1.49635893333199,1.6803005512817,133.85));
#44781=CARTESIAN_POINT('',(1.496358933332,1.68030055128166,132.6));
#44782=CARTESIAN_POINT('',(1.52027957955108,1.52027957955108,132.6));
#44783=CARTESIAN_POINT('',(1.496358933332,1.68030055128168,133.225));
#44784=CARTESIAN_POINT('Origin',(1.6142828459501,1.6142828459501,132.6));
#44785=CARTESIAN_POINT('Origin',(0.,0.,132.6));
#44786=CARTESIAN_POINT('Origin',(2.25165373832146,0.417319353377018,134.));
#44787=CARTESIAN_POINT('',(2.20336243006892,0.455734573804467,132.6));
#44788=CARTESIAN_POINT('',(2.20336243006893,0.455734573804454,133.85));
#44789=CARTESIAN_POINT('',(2.20336243006893,0.455734573804454,133.225));
#44790=CARTESIAN_POINT('',(2.0767405265215,0.55646094697042,132.6));
#44791=CARTESIAN_POINT('',(2.25165373832146,0.417319353377018,132.6));
#44792=CARTESIAN_POINT('',(2.0767405265215,0.55646094697042,133.95));
#44793=CARTESIAN_POINT('',(2.0767405265215,0.55646094697042,134.));
#44794=CARTESIAN_POINT('Ctrl Pts',(2.20336243006895,0.45573457380444,133.85));
#44795=CARTESIAN_POINT('Ctrl Pts',(2.13861259302836,0.507242378263746,133.902974875989));
#44796=CARTESIAN_POINT('Ctrl Pts',(2.0767405265215,0.55646094697042,133.95));
#44797=CARTESIAN_POINT('Origin',(2.0767405265215,0.55646094697042,134.));
#44798=CARTESIAN_POINT('',(2.13603512508614,0.707003496736936,133.85));
#44799=CARTESIAN_POINT('Ctrl Pts',(2.0767405265215,0.55646094697042,133.95));
#44800=CARTESIAN_POINT('Ctrl Pts',(2.10571402354757,0.630021511061296,133.902974875989));
#44801=CARTESIAN_POINT('Ctrl Pts',(2.13603512508614,0.707003496736956,133.85));
#44802=CARTESIAN_POINT('',(2.13603512508613,0.707003496736915,132.6));
#44803=CARTESIAN_POINT('',(2.0767405265215,0.55646094697042,132.6));
#44804=CARTESIAN_POINT('',(2.13603512508614,0.707003496736936,133.225));
#44805=CARTESIAN_POINT('Origin',(2.16419713242148,0.590868530511176,132.6));
#44806=CARTESIAN_POINT('Origin',(0.,0.,132.6));
#44807=CARTESIAN_POINT('Origin',(2.06692030116118,0.985870411690996,134.));
#44808=CARTESIAN_POINT('',(2.01033188866633,1.01047795493578,132.6));
#44809=CARTESIAN_POINT('',(2.01033188866635,1.01047795493577,133.85));
#44810=CARTESIAN_POINT('',(2.01033188866635,1.01047795493577,133.225));
#44811=CARTESIAN_POINT('',(1.86195461813654,1.075,132.6));
#44812=CARTESIAN_POINT('',(2.06692030116118,0.985870411690996,132.6));
#44813=CARTESIAN_POINT('',(1.86195461813654,1.075,133.95));
#44814=CARTESIAN_POINT('',(1.86195461813654,1.075,134.));
#44815=CARTESIAN_POINT('Ctrl Pts',(2.01033188866637,1.01047795493577,133.85));
#44816=CARTESIAN_POINT('Ctrl Pts',(1.93445714805535,1.04347218252507,133.902974875989));
#44817=CARTESIAN_POINT('Ctrl Pts',(1.86195461813654,1.075,133.95));
#44818=CARTESIAN_POINT('Origin',(1.86195461813654,1.075,134.));
#44819=CARTESIAN_POINT('',(1.8802655232717,1.23575950815512,133.85));
#44820=CARTESIAN_POINT('Ctrl Pts',(1.86195461813654,1.075,133.95));
#44821=CARTESIAN_POINT('Ctrl Pts',(1.87090199223678,1.15355294148582,133.902974875989));
#44822=CARTESIAN_POINT('Ctrl Pts',(1.88026552327171,1.23575950815514,133.85));
#44823=CARTESIAN_POINT('',(1.8802655232717,1.2357595081551,132.6));
#44824=CARTESIAN_POINT('',(1.86195461813654,1.075,132.6));
#44825=CARTESIAN_POINT('',(1.8802655232717,1.23575950815512,133.225));
#44826=CARTESIAN_POINT('Origin',(1.96443745964886,1.14147034712443,132.6));
#44827=CARTESIAN_POINT('Origin',(0.,0.,132.6));
#44828=CARTESIAN_POINT('Origin',(1.29707028255787,1.88724897194442,134.));
#44829=CARTESIAN_POINT('',(1.2357595081551,1.8802655232717,132.6));
#44830=CARTESIAN_POINT('',(1.23575950815512,1.8802655232717,133.85));
#44831=CARTESIAN_POINT('',(1.23575950815512,1.8802655232717,133.225));
#44832=CARTESIAN_POINT('',(1.075,1.86195461813654,132.6));
#44833=CARTESIAN_POINT('',(1.29707028255787,1.88724897194442,132.6));
#44834=CARTESIAN_POINT('',(1.075,1.86195461813654,133.95));
#44835=CARTESIAN_POINT('',(1.075,1.86195461813654,134.));
#44836=CARTESIAN_POINT('Ctrl Pts',(1.23575950815514,1.88026552327171,133.85));
#44837=CARTESIAN_POINT('Ctrl Pts',(1.15355294148583,1.87090199223679,133.902974875989));
#44838=CARTESIAN_POINT('Ctrl Pts',(1.075,1.86195461813654,133.95));
#44839=CARTESIAN_POINT('Origin',(1.075,1.86195461813654,134.));
#44840=CARTESIAN_POINT('',(1.01047795493577,2.01033188866635,133.85));
#44841=CARTESIAN_POINT('Ctrl Pts',(1.075,1.86195461813654,133.95));
#44842=CARTESIAN_POINT('Ctrl Pts',(1.04347218252507,1.93445714805536,133.902974875989));
#44843=CARTESIAN_POINT('Ctrl Pts',(1.01047795493577,2.01033188866637,133.85));
#44844=CARTESIAN_POINT('',(1.01047795493578,2.01033188866633,132.6));
#44845=CARTESIAN_POINT('',(1.075,1.86195461813654,132.6));
#44846=CARTESIAN_POINT('',(1.01047795493577,2.01033188866635,133.225));
#44847=CARTESIAN_POINT('Origin',(1.14147034712443,1.96443745964886,132.6));
#44848=CARTESIAN_POINT('Origin',(0.,0.,132.6));
#44849=CARTESIAN_POINT('Origin',(0.179671329216765,2.28294069424886,134.));
#44850=CARTESIAN_POINT('',(0.13006636539463,2.24623746309088,132.6));
#44851=CARTESIAN_POINT('',(0.130066365394648,2.2462374630909,133.85));
#44852=CARTESIAN_POINT('',(0.130066365394648,2.2462374630909,133.225));
#44853=CARTESIAN_POINT('',(1.3164953090834E-16,2.15,132.6));
#44854=CARTESIAN_POINT('',(0.179671329216765,2.28294069424886,132.6));
#44855=CARTESIAN_POINT('',(1.3164953090834E-16,2.15,133.95));
#44856=CARTESIAN_POINT('',(1.3164953090834E-16,2.15,134.));
#44857=CARTESIAN_POINT('Ctrl Pts',(0.130066365394665,2.24623746309091,133.85));
#44858=CARTESIAN_POINT('Ctrl Pts',(0.0635551558186174,2.1970251240109,133.902974875989));
#44859=CARTESIAN_POINT('Ctrl Pts',(1.3164953090834E-16,2.15,133.95));
#44860=CARTESIAN_POINT('Origin',(1.3164953090834E-16,2.15,134.));
#44861=CARTESIAN_POINT('',(-0.130066365394647,2.2462374630909,133.85));
#44862=CARTESIAN_POINT('Ctrl Pts',(1.3164953090834E-16,2.15,133.95));
#44863=CARTESIAN_POINT('Ctrl Pts',(-0.0635551558186092,2.19702512401089,
133.902974875989));
#44864=CARTESIAN_POINT('Ctrl Pts',(-0.130066365394664,2.24623746309091,
133.85));
#44865=CARTESIAN_POINT('',(-0.13006636539463,2.24623746309088,132.6));
#44866=CARTESIAN_POINT('',(1.3164953090834E-16,2.15,132.6));
#44867=CARTESIAN_POINT('',(-0.130066365394647,2.2462374630909,133.225));
#44868=CARTESIAN_POINT('Origin',(1.38777878078145E-16,2.21647034712443,
132.6));
#44869=CARTESIAN_POINT('Origin',(0.,0.,132.6));
#44870=CARTESIAN_POINT('Origin',(-0.985870411690995,2.06692030116118,134.));
#44871=CARTESIAN_POINT('',(-1.01047795493578,2.01033188866633,132.6));
#44872=CARTESIAN_POINT('',(-1.01047795493577,2.01033188866635,133.85));
#44873=CARTESIAN_POINT('',(-1.01047795493577,2.01033188866635,133.225));
#44874=CARTESIAN_POINT('',(-1.075,1.86195461813654,132.6));
#44875=CARTESIAN_POINT('',(-0.985870411690995,2.06692030116118,132.6));
#44876=CARTESIAN_POINT('',(-1.075,1.86195461813654,133.95));
#44877=CARTESIAN_POINT('',(-1.075,1.86195461813654,134.));
#44878=CARTESIAN_POINT('Ctrl Pts',(-1.01047795493577,2.01033188866637,133.85));
#44879=CARTESIAN_POINT('Ctrl Pts',(-1.04347218252506,1.93445714805537,133.902974875989));
#44880=CARTESIAN_POINT('Ctrl Pts',(-1.075,1.86195461813654,133.95));
#44881=CARTESIAN_POINT('Origin',(-1.075,1.86195461813654,134.));
#44882=CARTESIAN_POINT('',(-1.23575950815512,1.8802655232717,133.85));
#44883=CARTESIAN_POINT('Ctrl Pts',(-1.075,1.86195461813654,133.95));
#44884=CARTESIAN_POINT('Ctrl Pts',(-1.15355294148585,1.87090199223679,133.902974875989));
#44885=CARTESIAN_POINT('Ctrl Pts',(-1.23575950815514,1.88026552327171,133.85));
#44886=CARTESIAN_POINT('',(-1.2357595081551,1.8802655232717,132.6));
#44887=CARTESIAN_POINT('',(-1.075,1.86195461813654,132.6));
#44888=CARTESIAN_POINT('',(-1.23575950815512,1.8802655232717,133.225));
#44889=CARTESIAN_POINT('Origin',(-1.14147034712443,1.96443745964886,132.6));
#44890=CARTESIAN_POINT('Origin',(0.,0.,132.6));
#44891=CARTESIAN_POINT('Origin',(-1.88724897194442,1.29707028255787,134.));
#44892=CARTESIAN_POINT('',(-1.8802655232717,1.2357595081551,132.6));
#44893=CARTESIAN_POINT('',(-1.8802655232717,1.23575950815512,133.85));
#44894=CARTESIAN_POINT('',(-1.8802655232717,1.23575950815512,133.225));
#44895=CARTESIAN_POINT('',(-1.86195461813654,1.075,132.6));
#44896=CARTESIAN_POINT('',(-1.88724897194442,1.29707028255787,132.6));
#44897=CARTESIAN_POINT('',(-1.86195461813654,1.075,133.95));
#44898=CARTESIAN_POINT('',(-1.86195461813654,1.075,134.));
#44899=CARTESIAN_POINT('Ctrl Pts',(-1.88026552327171,1.23575950815514,133.85));
#44900=CARTESIAN_POINT('Ctrl Pts',(-1.87090199223678,1.1535529414858,133.902974875989));
#44901=CARTESIAN_POINT('Ctrl Pts',(-1.86195461813654,1.075,133.95));
#44902=CARTESIAN_POINT('Origin',(-1.86195461813654,1.075,134.));
#44903=CARTESIAN_POINT('',(-2.01033188866635,1.01047795493577,133.85));
#44904=CARTESIAN_POINT('Ctrl Pts',(-1.86195461813654,1.075,133.95));
#44905=CARTESIAN_POINT('Ctrl Pts',(-1.93445714805534,1.04347218252508,133.902974875989));
#44906=CARTESIAN_POINT('Ctrl Pts',(-2.01033188866637,1.01047795493577,133.85));
#44907=CARTESIAN_POINT('',(-2.01033188866633,1.01047795493578,132.6));
#44908=CARTESIAN_POINT('',(-1.86195461813654,1.075,132.6));
#44909=CARTESIAN_POINT('',(-2.01033188866635,1.01047795493577,133.225));
#44910=CARTESIAN_POINT('Origin',(-1.96443745964886,1.14147034712443,132.6));
#44911=CARTESIAN_POINT('Origin',(0.,0.,132.6));
#44912=CARTESIAN_POINT('Origin',(2.28294069424886,-0.179671329216765,134.));
#44913=CARTESIAN_POINT('',(2.24623746309088,-0.13006636539463,132.6));
#44914=CARTESIAN_POINT('',(2.2462374630909,-0.130066365394648,133.85));
#44915=CARTESIAN_POINT('',(2.2462374630909,-0.130066365394648,133.225));
#44916=CARTESIAN_POINT('',(2.15,0.,132.6));
#44917=CARTESIAN_POINT('',(2.28294069424886,-0.179671329216765,132.6));
#44918=CARTESIAN_POINT('',(2.15,0.,133.95));
#44919=CARTESIAN_POINT('',(2.15,0.,134.));
#44920=CARTESIAN_POINT('Ctrl Pts',(2.24623746309091,-0.130066365394665,
133.85));
#44921=CARTESIAN_POINT('Ctrl Pts',(2.19702512401089,-0.06355515581861,133.902974875989));
#44922=CARTESIAN_POINT('Ctrl Pts',(2.15,0.,133.95));
#44923=CARTESIAN_POINT('Origin',(2.15,0.,134.));
#44924=CARTESIAN_POINT('',(2.2462374630909,0.130066365394648,133.85));
#44925=CARTESIAN_POINT('Ctrl Pts',(2.15,0.,133.95));
#44926=CARTESIAN_POINT('Ctrl Pts',(2.19702512401088,0.0635551558185882,
133.902974875989));
#44927=CARTESIAN_POINT('Ctrl Pts',(2.24623746309091,0.130066365394665,133.85));
#44928=CARTESIAN_POINT('',(2.24623746309088,0.13006636539463,132.6));
#44929=CARTESIAN_POINT('',(2.15,0.,132.6));
#44930=CARTESIAN_POINT('',(2.2462374630909,0.130066365394648,133.225));
#44931=CARTESIAN_POINT('Origin',(2.21647034712443,0.,132.6));
#44932=CARTESIAN_POINT('Origin',(0.,0.,132.6));
#44933=CARTESIAN_POINT('Origin',(-2.25165373832146,-0.417319353377018,134.));
#44934=CARTESIAN_POINT('',(-2.20336243006892,-0.455734573804467,132.6));
#44935=CARTESIAN_POINT('',(-2.20336243006893,-0.455734573804454,133.85));
#44936=CARTESIAN_POINT('',(-2.20336243006893,-0.455734573804454,133.225));
#44937=CARTESIAN_POINT('',(-2.0767405265215,-0.55646094697042,132.6));
#44938=CARTESIAN_POINT('',(-2.25165373832146,-0.417319353377018,132.6));
#44939=CARTESIAN_POINT('',(-2.0767405265215,-0.55646094697042,133.95));
#44940=CARTESIAN_POINT('',(-2.0767405265215,-0.55646094697042,134.));
#44941=CARTESIAN_POINT('Ctrl Pts',(-2.20336243006895,-0.455734573804441,
133.85));
#44942=CARTESIAN_POINT('Ctrl Pts',(-2.13861259302836,-0.50724237826374,
133.902974875989));
#44943=CARTESIAN_POINT('Ctrl Pts',(-2.0767405265215,-0.55646094697042,133.95));
#44944=CARTESIAN_POINT('Origin',(-2.0767405265215,-0.55646094697042,134.));
#44945=CARTESIAN_POINT('',(-2.13603512508614,-0.707003496736936,133.85));
#44946=CARTESIAN_POINT('Ctrl Pts',(-2.0767405265215,-0.55646094697042,133.95));
#44947=CARTESIAN_POINT('Ctrl Pts',(-2.10571402354757,-0.630021511061296,
133.902974875989));
#44948=CARTESIAN_POINT('Ctrl Pts',(-2.13603512508614,-0.707003496736956,
133.85));
#44949=CARTESIAN_POINT('',(-2.13603512508613,-0.707003496736915,132.6));
#44950=CARTESIAN_POINT('',(-2.0767405265215,-0.55646094697042,132.6));
#44951=CARTESIAN_POINT('',(-2.13603512508614,-0.707003496736936,133.225));
#44952=CARTESIAN_POINT('Origin',(-2.16419713242148,-0.590868530511177,132.6));
#44953=CARTESIAN_POINT('Origin',(0.,0.,132.6));
#44954=CARTESIAN_POINT('Origin',(-1.74132966122407,-1.48723603067612,134.));
#44955=CARTESIAN_POINT('',(-1.68030055128166,-1.496358933332,132.6));
#44956=CARTESIAN_POINT('',(-1.68030055128168,-1.496358933332,133.85));
#44957=CARTESIAN_POINT('',(-1.68030055128168,-1.496358933332,133.225));
#44958=CARTESIAN_POINT('',(-1.52027957955108,-1.52027957955108,132.6));
#44959=CARTESIAN_POINT('',(-1.74132966122407,-1.48723603067612,132.6));
#44960=CARTESIAN_POINT('',(-1.52027957955108,-1.52027957955108,133.95));
#44961=CARTESIAN_POINT('',(-1.52027957955108,-1.52027957955108,134.));
#44962=CARTESIAN_POINT('Ctrl Pts',(-1.6803005512817,-1.49635893333199,133.85));
#44963=CARTESIAN_POINT('Ctrl Pts',(-1.598471645284,-1.50859108196662,133.902974875989));
#44964=CARTESIAN_POINT('Ctrl Pts',(-1.52027957955108,-1.52027957955108,
133.95));
#44965=CARTESIAN_POINT('Origin',(-1.52027957955108,-1.52027957955108,134.));
#44966=CARTESIAN_POINT('',(-1.496358933332,-1.68030055128168,133.85));
#44967=CARTESIAN_POINT('Ctrl Pts',(-1.52027957955108,-1.52027957955108,
133.95));
#44968=CARTESIAN_POINT('Ctrl Pts',(-1.50859108196661,-1.59847164528404,
133.902974875989));
#44969=CARTESIAN_POINT('Ctrl Pts',(-1.49635893333199,-1.6803005512817,133.85));
#44970=CARTESIAN_POINT('',(-1.496358933332,-1.68030055128166,132.6));
#44971=CARTESIAN_POINT('',(-1.52027957955108,-1.52027957955108,132.6));
#44972=CARTESIAN_POINT('',(-1.496358933332,-1.68030055128168,133.225));
#44973=CARTESIAN_POINT('Origin',(-1.6142828459501,-1.6142828459501,132.6));
#44974=CARTESIAN_POINT('Origin',(0.,0.,132.6));
#44975=CARTESIAN_POINT('Origin',(-0.764417707645336,-2.15864901460109,134.));
#44976=CARTESIAN_POINT('',(-0.707003496736916,-2.13603512508613,132.6));
#44977=CARTESIAN_POINT('',(-0.707003496736936,-2.13603512508614,133.85));
#44978=CARTESIAN_POINT('',(-0.707003496736936,-2.13603512508614,133.225));
#44979=CARTESIAN_POINT('',(-0.556460946970419,-2.0767405265215,132.6));
#44980=CARTESIAN_POINT('',(-0.764417707645336,-2.15864901460109,132.6));
#44981=CARTESIAN_POINT('',(-0.556460946970419,-2.0767405265215,133.95));
#44982=CARTESIAN_POINT('',(-0.556460946970419,-2.0767405265215,134.));
#44983=CARTESIAN_POINT('Ctrl Pts',(-0.707003496736956,-2.13603512508614,
133.85));
#44984=CARTESIAN_POINT('Ctrl Pts',(-0.630021511061715,-2.10571402354773,
133.902974875989));
#44985=CARTESIAN_POINT('Ctrl Pts',(-0.556460946970419,-2.0767405265215,
133.95));
#44986=CARTESIAN_POINT('Origin',(-0.556460946970419,-2.0767405265215,134.));
#44987=CARTESIAN_POINT('',(-0.455734573804454,-2.20336243006893,133.85));
#44988=CARTESIAN_POINT('Ctrl Pts',(-0.556460946970419,-2.0767405265215,
133.95));
#44989=CARTESIAN_POINT('Ctrl Pts',(-0.507242378263734,-2.13861259302837,
133.902974875989));
#44990=CARTESIAN_POINT('Ctrl Pts',(-0.455734573804441,-2.20336243006895,
133.85));
#44991=CARTESIAN_POINT('',(-0.455734573804468,-2.20336243006892,132.6));
#44992=CARTESIAN_POINT('',(-0.556460946970419,-2.0767405265215,132.6));
#44993=CARTESIAN_POINT('',(-0.455734573804454,-2.20336243006893,133.225));
#44994=CARTESIAN_POINT('Origin',(-0.590868530511177,-2.16419713242148,132.6));
#44995=CARTESIAN_POINT('Origin',(0.,0.,132.6));
#44996=CARTESIAN_POINT('Origin',(0.417319353377018,-2.25165373832146,134.));
#44997=CARTESIAN_POINT('',(0.455734573804467,-2.20336243006892,132.6));
#44998=CARTESIAN_POINT('',(0.455734573804453,-2.20336243006893,133.85));
#44999=CARTESIAN_POINT('',(0.455734573804453,-2.20336243006893,133.225));
#45000=CARTESIAN_POINT('',(0.556460946970419,-2.0767405265215,132.6));
#45001=CARTESIAN_POINT('',(0.417319353377018,-2.25165373832146,132.6));
#45002=CARTESIAN_POINT('',(0.556460946970419,-2.0767405265215,133.95));
#45003=CARTESIAN_POINT('',(0.556460946970419,-2.0767405265215,134.));
#45004=CARTESIAN_POINT('Ctrl Pts',(0.45573457380444,-2.20336243006895,133.85));
#45005=CARTESIAN_POINT('Ctrl Pts',(0.507242378263739,-2.13861259302836,
133.902974875989));
#45006=CARTESIAN_POINT('Ctrl Pts',(0.556460946970419,-2.0767405265215,133.95));
#45007=CARTESIAN_POINT('Origin',(0.556460946970419,-2.0767405265215,134.));
#45008=CARTESIAN_POINT('',(0.707003496736935,-2.13603512508614,133.85));
#45009=CARTESIAN_POINT('Ctrl Pts',(0.556460946970419,-2.0767405265215,133.95));
#45010=CARTESIAN_POINT('Ctrl Pts',(0.630021511061762,-2.10571402354775,
133.902974875989));
#45011=CARTESIAN_POINT('Ctrl Pts',(0.707003496736956,-2.13603512508614,
133.85));
#45012=CARTESIAN_POINT('',(0.707003496736915,-2.13603512508613,132.6));
#45013=CARTESIAN_POINT('',(0.556460946970419,-2.0767405265215,132.6));
#45014=CARTESIAN_POINT('',(0.707003496736935,-2.13603512508614,133.225));
#45015=CARTESIAN_POINT('Origin',(0.590868530511176,-2.16419713242148,132.6));
#45016=CARTESIAN_POINT('Origin',(0.,0.,132.6));
#45017=CARTESIAN_POINT('Origin',(1.48723603067612,-1.74132966122407,134.));
#45018=CARTESIAN_POINT('',(1.496358933332,-1.68030055128166,132.6));
#45019=CARTESIAN_POINT('',(1.496358933332,-1.68030055128168,133.85));
#45020=CARTESIAN_POINT('',(1.496358933332,-1.68030055128168,133.225));
#45021=CARTESIAN_POINT('',(1.52027957955108,-1.52027957955108,132.6));
#45022=CARTESIAN_POINT('',(1.48723603067612,-1.74132966122407,132.6));
#45023=CARTESIAN_POINT('',(1.52027957955108,-1.52027957955108,133.95));
#45024=CARTESIAN_POINT('',(1.52027957955108,-1.52027957955108,134.));
#45025=CARTESIAN_POINT('Ctrl Pts',(1.49635893333199,-1.6803005512817,133.85));
#45026=CARTESIAN_POINT('Ctrl Pts',(1.50859108196662,-1.59847164528399,133.902974875989));
#45027=CARTESIAN_POINT('Ctrl Pts',(1.52027957955108,-1.52027957955108,133.95));
#45028=CARTESIAN_POINT('Origin',(1.52027957955108,-1.52027957955108,134.));
#45029=CARTESIAN_POINT('',(1.68030055128168,-1.496358933332,133.85));
#45030=CARTESIAN_POINT('Ctrl Pts',(1.52027957955108,-1.52027957955108,133.95));
#45031=CARTESIAN_POINT('Ctrl Pts',(1.59847164528402,-1.50859108196661,133.902974875989));
#45032=CARTESIAN_POINT('Ctrl Pts',(1.6803005512817,-1.49635893333199,133.85));
#45033=CARTESIAN_POINT('',(1.68030055128166,-1.496358933332,132.6));
#45034=CARTESIAN_POINT('',(1.52027957955108,-1.52027957955108,132.6));
#45035=CARTESIAN_POINT('',(1.68030055128168,-1.496358933332,133.225));
#45036=CARTESIAN_POINT('Origin',(1.6142828459501,-1.6142828459501,132.6));
#45037=CARTESIAN_POINT('Origin',(0.,0.,132.6));
#45038=CARTESIAN_POINT('Origin',(2.15864901460109,-0.764417707645336,134.));
#45039=CARTESIAN_POINT('',(2.13603512508613,-0.707003496736916,132.6));
#45040=CARTESIAN_POINT('',(2.13603512508614,-0.707003496736936,133.85));
#45041=CARTESIAN_POINT('',(2.13603512508614,-0.707003496736936,133.225));
#45042=CARTESIAN_POINT('',(2.0767405265215,-0.556460946970419,132.6));
#45043=CARTESIAN_POINT('',(2.15864901460109,-0.764417707645336,132.6));
#45044=CARTESIAN_POINT('',(2.0767405265215,-0.556460946970419,133.95));
#45045=CARTESIAN_POINT('',(2.0767405265215,-0.556460946970419,134.));
#45046=CARTESIAN_POINT('Ctrl Pts',(2.13603512508614,-0.707003496736956,
133.85));
#45047=CARTESIAN_POINT('Ctrl Pts',(2.10571402354774,-0.630021511061738,
133.902974875989));
#45048=CARTESIAN_POINT('Ctrl Pts',(2.0767405265215,-0.556460946970419,133.95));
#45049=CARTESIAN_POINT('Origin',(2.0767405265215,-0.556460946970419,134.));
#45050=CARTESIAN_POINT('',(2.20336243006893,-0.455734573804454,133.85));
#45051=CARTESIAN_POINT('Ctrl Pts',(2.0767405265215,-0.556460946970419,133.95));
#45052=CARTESIAN_POINT('Ctrl Pts',(2.13861259302834,-0.507242378263754,
133.902974875989));
#45053=CARTESIAN_POINT('Ctrl Pts',(2.20336243006895,-0.455734573804441,
133.85));
#45054=CARTESIAN_POINT('',(2.20336243006892,-0.455734573804468,132.6));
#45055=CARTESIAN_POINT('',(2.0767405265215,-0.556460946970419,132.6));
#45056=CARTESIAN_POINT('',(2.20336243006893,-0.455734573804454,133.225));
#45057=CARTESIAN_POINT('Origin',(2.16419713242148,-0.590868530511177,132.6));
#45058=CARTESIAN_POINT('Origin',(0.,0.,132.6));
#45059=CARTESIAN_POINT('Origin',(0.,0.,133.925));
#45060=CARTESIAN_POINT('',(-2.10000000000001,-2.57175827820945E-16,134.));
#45061=CARTESIAN_POINT('Origin',(0.,0.,134.));
#45062=CARTESIAN_POINT('',(-2.175,-2.66360678814549E-16,133.925));
#45063=CARTESIAN_POINT('Origin',(0.,0.,133.85));
#45064=CARTESIAN_POINT('Origin',(0.,0.,133.85));
#45065=CARTESIAN_POINT('Origin',(0.,0.,133.85));
#45066=CARTESIAN_POINT('Origin',(0.,0.,133.85));
#45067=CARTESIAN_POINT('Origin',(0.,0.,133.85));
#45068=CARTESIAN_POINT('Origin',(0.,0.,133.85));
#45069=CARTESIAN_POINT('Origin',(0.,0.,133.85));
#45070=CARTESIAN_POINT('Origin',(0.,0.,133.85));
#45071=CARTESIAN_POINT('Origin',(0.,0.,133.85));
#45072=CARTESIAN_POINT('Origin',(0.,0.,133.85));
#45073=CARTESIAN_POINT('Origin',(0.,0.,133.85));
#45074=CARTESIAN_POINT('Origin',(0.,0.,133.85));
#45075=CARTESIAN_POINT('Origin',(0.,0.,133.85));
#45076=CARTESIAN_POINT('Origin',(0.,0.,133.85));
#45077=CARTESIAN_POINT('Origin',(0.,0.,133.85));
#45078=CARTESIAN_POINT('Origin',(0.,0.,133.85));
#45079=CARTESIAN_POINT('Origin',(0.,0.,133.85));
#45080=CARTESIAN_POINT('Origin',(0.,0.,133.85));
#45081=CARTESIAN_POINT('Origin',(0.,0.,133.85));
#45082=CARTESIAN_POINT('Origin',(0.,0.,133.85));
#45083=CARTESIAN_POINT('Origin',(0.,0.,133.85));
#45084=CARTESIAN_POINT('Origin',(0.,0.,133.85));
#45085=CARTESIAN_POINT('Origin',(0.,0.,133.85));
#45086=CARTESIAN_POINT('Origin',(0.,0.,133.85));
#45087=CARTESIAN_POINT('Origin',(0.,0.,133.225));
#45088=CARTESIAN_POINT('Origin',(0.,0.,132.6));
#45089=CARTESIAN_POINT('Origin',(0.,0.,133.225));
#45090=CARTESIAN_POINT('Origin',(0.,0.,132.6));
#45091=CARTESIAN_POINT('Origin',(0.,0.,133.225));
#45092=CARTESIAN_POINT('Origin',(0.,0.,132.6));
#45093=CARTESIAN_POINT('Origin',(0.,0.,133.225));
#45094=CARTESIAN_POINT('Origin',(0.,0.,132.6));
#45095=CARTESIAN_POINT('Origin',(0.,0.,133.225));
#45096=CARTESIAN_POINT('Origin',(0.,0.,132.6));
#45097=CARTESIAN_POINT('Origin',(0.,0.,133.225));
#45098=CARTESIAN_POINT('Origin',(0.,0.,132.6));
#45099=CARTESIAN_POINT('Origin',(0.,0.,133.225));
#45100=CARTESIAN_POINT('Origin',(0.,0.,132.6));
#45101=CARTESIAN_POINT('Origin',(0.,0.,133.225));
#45102=CARTESIAN_POINT('Origin',(0.,0.,132.6));
#45103=CARTESIAN_POINT('Origin',(0.,0.,133.225));
#45104=CARTESIAN_POINT('Origin',(0.,0.,132.6));
#45105=CARTESIAN_POINT('Origin',(0.,0.,133.225));
#45106=CARTESIAN_POINT('Origin',(0.,0.,132.6));
#45107=CARTESIAN_POINT('Origin',(0.,0.,133.225));
#45108=CARTESIAN_POINT('Origin',(0.,0.,132.6));
#45109=CARTESIAN_POINT('Origin',(0.,0.,133.225));
#45110=CARTESIAN_POINT('Origin',(0.,0.,132.6));
#45111=CARTESIAN_POINT('Origin',(0.,0.,133.225));
#45112=CARTESIAN_POINT('Origin',(0.,0.,132.6));
#45113=CARTESIAN_POINT('Origin',(0.,0.,133.225));
#45114=CARTESIAN_POINT('Origin',(0.,0.,132.6));
#45115=CARTESIAN_POINT('Origin',(0.,0.,133.225));
#45116=CARTESIAN_POINT('Origin',(0.,0.,132.6));
#45117=CARTESIAN_POINT('Origin',(0.,0.,133.225));
#45118=CARTESIAN_POINT('Origin',(0.,0.,132.6));
#45119=CARTESIAN_POINT('Origin',(0.,0.,133.225));
#45120=CARTESIAN_POINT('Origin',(0.,0.,132.6));
#45121=CARTESIAN_POINT('Origin',(0.,0.,133.225));
#45122=CARTESIAN_POINT('Origin',(0.,0.,132.6));
#45123=CARTESIAN_POINT('Origin',(0.,0.,133.225));
#45124=CARTESIAN_POINT('Origin',(0.,0.,132.6));
#45125=CARTESIAN_POINT('Origin',(0.,0.,133.225));
#45126=CARTESIAN_POINT('Origin',(0.,0.,132.6));
#45127=CARTESIAN_POINT('Origin',(0.,0.,133.225));
#45128=CARTESIAN_POINT('Origin',(0.,0.,132.6));
#45129=CARTESIAN_POINT('Origin',(0.,0.,133.225));
#45130=CARTESIAN_POINT('Origin',(0.,0.,132.6));
#45131=CARTESIAN_POINT('Origin',(0.,0.,133.225));
#45132=CARTESIAN_POINT('Origin',(0.,0.,132.6));
#45133=CARTESIAN_POINT('Ctrl Pts',(-0.557371730700663,1.15960179105404,
130.884457777378));
#45134=CARTESIAN_POINT('Ctrl Pts',(-0.744210289770409,1.06979636661117,
130.893433011949));
#45135=CARTESIAN_POINT('Ctrl Pts',(-1.07348944454164,0.798225397208331,
130.911383481089));
#45136=CARTESIAN_POINT('Ctrl Pts',(-1.32154880708789,0.207818302348253,
130.938309184799));
#45137=CARTESIAN_POINT('Ctrl Pts',(-1.2667357611315,-0.430175148668094,
130.96523488851));
#45138=CARTESIAN_POINT('Ctrl Pts',(-0.921694221117689,-0.969633149057105,
130.99216059222));
#45139=CARTESIAN_POINT('Ctrl Pts',(-0.365449910586059,-1.28691209396646,
131.01908629593));
#45140=CARTESIAN_POINT('Ctrl Pts',(0.274526574308514,-1.30932546829921,
131.046011999641));
#45141=CARTESIAN_POINT('Ctrl Pts',(0.851603122293372,-1.03172996338952,
131.072937703351));
#45142=CARTESIAN_POINT('Ctrl Pts',(1.23354957705434,-0.517733871181562,
131.099863407061));
#45143=CARTESIAN_POINT('Ctrl Pts',(1.3328512265448,0.114891597751729,131.126789110772));
#45144=CARTESIAN_POINT('Ctrl Pts',(1.12675416518279,0.721191403089574,131.153714814482));
#45145=CARTESIAN_POINT('Ctrl Pts',(0.662482047549443,1.16224333958056,131.180640518192));
#45146=CARTESIAN_POINT('Ctrl Pts',(0.0464142156206867,1.33698831153762,
131.207566221903));
#45147=CARTESIAN_POINT('Ctrl Pts',(-0.580288559487598,1.20538676777764,
131.234491925613));
#45148=CARTESIAN_POINT('Ctrl Pts',(-1.07402878803166,0.797592790182427,
131.261417629323));
#45149=CARTESIAN_POINT('Ctrl Pts',(-1.32167488266001,0.207044955006741,
131.288343333034));
#45150=CARTESIAN_POINT('Ctrl Pts',(-1.26648325984221,-0.430943463576776,
131.315269036744));
#45151=CARTESIAN_POINT('Ctrl Pts',(-0.92110007241593,-0.970189040198561,
131.342194740455));
#45152=CARTESIAN_POINT('Ctrl Pts',(-0.364663586223146,-1.28713347653886,
131.369120444165));
#45153=CARTESIAN_POINT('Ctrl Pts',(0.275328916768196,-1.30915472904038,
131.396046147875));
#45154=CARTESIAN_POINT('Ctrl Pts',(0.852234815095578,-1.03120702894802,
131.422971851586));
#45155=CARTESIAN_POINT('Ctrl Pts',(1.23386663366973,-0.516977027235267,
131.449897555296));
#45156=CARTESIAN_POINT('Ctrl Pts',(1.332780394676,0.115708840682625,131.476823259006));
#45157=CARTESIAN_POINT('Ctrl Pts',(1.1263118120373,0.721882135998308,131.503748962717));
#45158=CARTESIAN_POINT('Ctrl Pts',(0.661769399512303,1.16264929280748,131.530674666427));
#45159=CARTESIAN_POINT('Ctrl Pts',(0.0455945867891589,1.33701654808655,
131.557600370137));
#45160=CARTESIAN_POINT('Ctrl Pts',(-0.581027394744716,1.20503082232908,
131.584526073848));
#45161=CARTESIAN_POINT('Ctrl Pts',(-1.07451753531689,0.796934239763604,
131.611451777558));
#45162=CARTESIAN_POINT('Ctrl Pts',(-1.32180156079828,0.206234696607059,
131.638377481268));
#45163=CARTESIAN_POINT('Ctrl Pts',(-1.26621884236099,-0.431719769601012,
131.665303184979));
#45164=CARTESIAN_POINT('Ctrl Pts',(-0.920505147196365,-0.970753516707333,
131.692228888689));
#45165=CARTESIAN_POINT('Ctrl Pts',(-0.363874469513489,-1.2873567829668,
131.7191545924));
#45166=CARTESIAN_POINT('Ctrl Pts',(0.276131412923829,-1.30898569855063,
131.74608029611));
#45167=CARTESIAN_POINT('Ctrl Pts',(0.852866813310974,-1.03068439153984,
131.77300599982));
#45168=CARTESIAN_POINT('Ctrl Pts',(1.23418332299191,-0.516220535677922,
131.799931703531));
#45169=CARTESIAN_POINT('Ctrl Pts',(1.33270921150778,0.116525850196642,131.826857407241));
#45170=CARTESIAN_POINT('Ctrl Pts',(1.12586906668276,0.722572460645641,131.853783110951));
#45171=CARTESIAN_POINT('Ctrl Pts',(0.661056538993872,1.16305475729291,131.880708814662));
#45172=CARTESIAN_POINT('Ctrl Pts',(0.0447749500858785,1.33704424761847,
131.907634518372));
#45173=CARTESIAN_POINT('Ctrl Pts',(-0.581766002838075,1.20467441008527,
131.934560222082));
#45174=CARTESIAN_POINT('Ctrl Pts',(-1.07500587627816,0.796275381121529,
131.961485925793));
#45175=CARTESIAN_POINT('Ctrl Pts',(-1.32192774026812,0.205424357093238,
131.988411629503));
#45176=CARTESIAN_POINT('Ctrl Pts',(-1.26595394887095,-0.432495915451445,
132.015337333214));
#45177=CARTESIAN_POINT('Ctrl Pts',(-0.919909876517952,-0.971317628899406,
132.042263036924));
#45178=CARTESIAN_POINT('Ctrl Pts',(-0.363085218132085,-1.28757960555225,
132.069188740634));
#45179=CARTESIAN_POINT('Ctrl Pts',(0.276933801600455,-1.30881617440312,
132.096114444345));
#45180=CARTESIAN_POINT('Ctrl Pts',(0.853498482162152,-1.0301613647476,132.123040148055));
#45181=CARTESIAN_POINT('Ctrl Pts',(1.23449953411498,-0.51546384206413,132.149965851765));
#45182=CARTESIAN_POINT('Ctrl Pts',(1.33263749249817,0.117342823334407,132.176891555476));
#45183=CARTESIAN_POINT('Ctrl Pts',(1.125425844559,0.72326254715928,132.203817259186));
#45184=CARTESIAN_POINT('Ctrl Pts',(0.660343291616316,1.16345980844394,132.230742962896));
#45185=CARTESIAN_POINT('Ctrl Pts',(0.0439550989490249,1.33707158395214,
132.257668666607));
#45186=CARTESIAN_POINT('Ctrl Pts',(-0.582504943319958,1.20431761235457,
132.284594370317));
#45187=CARTESIAN_POINT('Ctrl Pts',(-1.07549453007113,0.795616811689296,
132.311520074027));
#45188=CARTESIAN_POINT('Ctrl Pts',(-1.32205563425755,0.204614080322882,
132.338445777738));
#45189=CARTESIAN_POINT('Ctrl Pts',(-1.2656911247959,-0.43326937505133,132.365371481448));
#45190=CARTESIAN_POINT('Ctrl Pts',(-0.919323220327711,-0.971881421552252,
132.392297185159));
#45191=CARTESIAN_POINT('Ctrl Pts',(-0.362304579342239,-1.28779095308542,
132.419222888869));
#45192=CARTESIAN_POINT('Ctrl Pts',(0.277699363289323,-1.30864921194912,
132.446148592579));
#45193=CARTESIAN_POINT('Ctrl Pts',(0.85410155756253,-1.02958919072608,132.47307429629));
#45194=CARTESIAN_POINT('Ctrl Pts',(1.10780466901396,-0.686354162750902,
132.49102476543));
#45195=CARTESIAN_POINT('Ctrl Pts',(1.18756226708949,-0.495010526943894,
132.5));
#45196=CARTESIAN_POINT('Ctrl Pts',(-0.586270641941264,1.21972545249627,
130.922971851586));
#45197=CARTESIAN_POINT('Ctrl Pts',(-0.78279650777142,1.12526374778845,130.931947086156));
#45198=CARTESIAN_POINT('Ctrl Pts',(-1.1291483064228,0.839612219742223,130.949897555296));
#45199=CARTESIAN_POINT('Ctrl Pts',(-1.39006918509154,0.21859337819608,130.976823259006));
#45200=CARTESIAN_POINT('Ctrl Pts',(-1.33241416265397,-0.452479102662395,
131.003748962717));
#45201=CARTESIAN_POINT('Ctrl Pts',(-0.969482722076592,-1.01990721350476,
131.030674666427));
#45202=CARTESIAN_POINT('Ctrl Pts',(-0.384397955395643,-1.35363660891672,
131.057600370137));
#45203=CARTESIAN_POINT('Ctrl Pts',(0.288760376755141,-1.37721208401592,
131.084526073848));
#45204=CARTESIAN_POINT('Ctrl Pts',(0.89575750201485,-1.08522365708435,131.111451777558));
#45205=CARTESIAN_POINT('Ctrl Pts',(1.29750732333861,-0.544577617222861,
131.138377481268));
#45206=CARTESIAN_POINT('Ctrl Pts',(1.40195761851129,0.120848559511423,131.165303184979));
#45207=CARTESIAN_POINT('Ctrl Pts',(1.18517472513595,0.758584125392103,131.192228888689));
#45208=CARTESIAN_POINT('Ctrl Pts',(0.696830775402138,1.22250396146085,131.2191545924));
#45209=CARTESIAN_POINT('Ctrl Pts',(0.0488207249996935,1.40630920532654,
131.24608029611));
#45210=CARTESIAN_POINT('Ctrl Pts',(-0.610375674873748,1.26788431347988,
131.27300599982));
#45211=CARTESIAN_POINT('Ctrl Pts',(-1.12971561408608,0.838946812964761,
131.299931703531));
#45212=CARTESIAN_POINT('Ctrl Pts',(-1.39020179749817,0.217779933922935,
131.326857407241));
#45213=CARTESIAN_POINT('Ctrl Pts',(-1.33214856954114,-0.453287253578409,
131.353783110951));
#45214=CARTESIAN_POINT('Ctrl Pts',(-0.968857767631288,-1.02049192679106,
131.380708814662));
#45215=CARTESIAN_POINT('Ctrl Pts',(-0.383570861261465,-1.35386946985259,
131.407634518372));
#45216=CARTESIAN_POINT('Ctrl Pts',(0.28960431950104,-1.37703249217557,131.434560222082));
#45217=CARTESIAN_POINT('Ctrl Pts',(0.896421947167448,-1.08467360925483,
131.461485925793));
#45218=CARTESIAN_POINT('Ctrl Pts',(1.29784081887703,-0.543781532021902,
131.488411629503));
#45219=CARTESIAN_POINT('Ctrl Pts',(1.40188311411341,0.121708175296234,131.515337333214));
#45220=CARTESIAN_POINT('Ctrl Pts',(1.1847094366251,0.759310671794635,131.542263036924));
#45221=CARTESIAN_POINT('Ctrl Pts',(0.696081177603758,1.22293096277045,131.569188740634));
#45222=CARTESIAN_POINT('Ctrl Pts',(0.047958599608781,1.40633890589934,131.596114444345));
#45223=CARTESIAN_POINT('Ctrl Pts',(-0.611152817661263,1.26750991277901,
131.623040148055));
#45224=CARTESIAN_POINT('Ctrl Pts',(-1.13022970220514,0.838254117667301,
131.649965851765));
#45225=CARTESIAN_POINT('Ctrl Pts',(-1.39033504371314,0.216927664807091,
131.676891555476));
#45226=CARTESIAN_POINT('Ctrl Pts',(-1.3318704423992,-0.454103809937662,
131.703817259186));
#45227=CARTESIAN_POINT('Ctrl Pts',(-0.968231996406861,-1.02108567058346,
131.730742962896));
#45228=CARTESIAN_POINT('Ctrl Pts',(-0.382740830001438,-1.3541043543931,
131.757668666607));
#45229=CARTESIAN_POINT('Ctrl Pts',(0.290448423911803,-1.37685469770148,
131.784594370317));
#45230=CARTESIAN_POINT('Ctrl Pts',(0.897086713568465,-1.08412387385937,
131.811520074027));
#45231=CARTESIAN_POINT('Ctrl Pts',(1.29817392807863,-0.542985817480746,
131.838445777738));
#45232=CARTESIAN_POINT('Ctrl Pts',(1.40180824020176,0.122567545561843,131.865371481448));
#45233=CARTESIAN_POINT('Ctrl Pts',(1.18424373556972,0.760036788768008,131.892297185159));
#45234=CARTESIAN_POINT('Ctrl Pts',(0.695331356307243,1.22335744999804,131.919222888869));
#45235=CARTESIAN_POINT('Ctrl Pts',(0.0470964659379791,1.40636804161159,
131.946148592579));
#45236=CARTESIAN_POINT('Ctrl Pts',(-0.611929721506911,1.26713502108022,
131.97307429629));
#45237=CARTESIAN_POINT('Ctrl Pts',(-1.13074336293295,0.837561098165661,
132.));
#45238=CARTESIAN_POINT('Ctrl Pts',(-1.39046776540444,0.216075310371461,
132.02692570371));
#45239=CARTESIAN_POINT('Ctrl Pts',(-1.33159181456808,-0.454920197818335,
132.053851407421));
#45240=CARTESIAN_POINT('Ctrl Pts',(-0.967605861812048,-1.02167903116986,
132.080777111131));
#45241=CARTESIAN_POINT('Ctrl Pts',(-0.38191065708713,-1.35433873000459,
132.107702814841));
#45242=CARTESIAN_POINT('Ctrl Pts',(0.291292415270928,-1.37667638397419,
132.134628518552));
#45243=CARTESIAN_POINT('Ctrl Pts',(0.897751133528208,-1.08357372889085,
132.161554222262));
#45244=CARTESIAN_POINT('Ctrl Pts',(1.29850653428721,-0.542189890406811,
132.188479925973));
#45245=CARTESIAN_POINT('Ctrl Pts',(1.40173280266611,0.123426877565145,132.215405629683));
#45246=CARTESIAN_POINT('Ctrl Pts',(1.18377753302534,0.760762655260802,132.242331333393));
#45247=CARTESIAN_POINT('Ctrl Pts',(0.69458112809352,1.22378350246043,132.269257037104));
#45248=CARTESIAN_POINT('Ctrl Pts',(0.046234106715534,1.40639679529429,132.296182740814));
#45249=CARTESIAN_POINT('Ctrl Pts',(-0.612706974974943,1.26675972390762,
132.323108444524));
#45250=CARTESIAN_POINT('Ctrl Pts',(-1.13125735271232,0.836868382868973,
132.350034148235));
#45251=CARTESIAN_POINT('Ctrl Pts',(-1.39060229051067,0.215223021932451,
132.376959851945));
#45252=CARTESIAN_POINT('Ctrl Pts',(-1.33131536344811,-0.455733760170286,
132.403885555655));
#45253=CARTESIAN_POINT('Ctrl Pts',(-0.966988788354056,-1.02227205564939,
132.430811259366));
#45254=CARTESIAN_POINT('Ctrl Pts',(-0.381089543314689,-1.35456103559908,
132.457736963076));
#45255=CARTESIAN_POINT('Ctrl Pts',(0.292097670216696,-1.37650076476049,
132.484662666786));
#45256=CARTESIAN_POINT('Ctrl Pts',(0.898385477508435,-1.0829718884809,132.511588370497));
#45257=CARTESIAN_POINT('Ctrl Pts',(1.16524272523097,-0.721940624956333,
132.529538839637));
#45258=CARTESIAN_POINT('Ctrl Pts',(1.24913563843031,-0.520676100731304,
132.538514074207));
#45259=CARTESIAN_POINT('Ctrl Pts',(-0.615169553181865,1.27984911393849,
130.961485925793));
#45260=CARTESIAN_POINT('Ctrl Pts',(-0.821382725772432,1.18073112896573,
130.970461160363));
#45261=CARTESIAN_POINT('Ctrl Pts',(-1.18480716830396,0.880999042276115,
130.988411629503));
#45262=CARTESIAN_POINT('Ctrl Pts',(-1.45858956309518,0.229368454043907,
131.015337333214));
#45263=CARTESIAN_POINT('Ctrl Pts',(-1.39809256417645,-0.474783056656697,
131.042263036924));
#45264=CARTESIAN_POINT('Ctrl Pts',(-1.0172712230355,-1.07018127795241,131.069188740634));
#45265=CARTESIAN_POINT('Ctrl Pts',(-0.403346000205227,-1.42036112386699,
131.096114444345));
#45266=CARTESIAN_POINT('Ctrl Pts',(0.30299417920177,-1.44509869973264,131.123040148055));
#45267=CARTESIAN_POINT('Ctrl Pts',(0.939911881736328,-1.13871735077919,
131.149965851765));
#45268=CARTESIAN_POINT('Ctrl Pts',(1.36146506962287,-0.571421363264162,
131.176891555476));
#45269=CARTESIAN_POINT('Ctrl Pts',(1.47106401047779,0.126805521271117,131.203817259186));
#45270=CARTESIAN_POINT('Ctrl Pts',(1.24359528508911,0.795976847694632,131.230742962896));
#45271=CARTESIAN_POINT('Ctrl Pts',(0.731179503254833,1.28276458334115,131.257668666607));
#45272=CARTESIAN_POINT('Ctrl Pts',(0.0512272343786986,1.47563009911546,
131.284594370317));
#45273=CARTESIAN_POINT('Ctrl Pts',(-0.640462790259896,1.33038185918212,
131.311520074028));
#45274=CARTESIAN_POINT('Ctrl Pts',(-1.18540244014049,0.880300835747097,
131.338445777738));
#45275=CARTESIAN_POINT('Ctrl Pts',(-1.45872871233634,0.228514912839127,
131.365371481448));
#45276=CARTESIAN_POINT('Ctrl Pts',(-1.39781387924007,-0.475631043580043,
131.392297185159));
#45277=CARTESIAN_POINT('Ctrl Pts',(-1.01661546284665,-1.07079481338356,
131.419222888869));
#45278=CARTESIAN_POINT('Ctrl Pts',(-0.402478136299785,-1.42060546316632,
131.446148592579));
#45279=CARTESIAN_POINT('Ctrl Pts',(0.303879722233887,-1.44491025531076,
131.47307429629));
#45280=CARTESIAN_POINT('Ctrl Pts',(0.940609079239318,-1.13814018956164,
131.5));
#45281=CARTESIAN_POINT('Ctrl Pts',(1.36181500408434,-0.570586036808538,
131.52692570371));
#45282=CARTESIAN_POINT('Ctrl Pts',(1.47098583355083,0.127707509909844,131.553851407421));
#45283=CARTESIAN_POINT('Ctrl Pts',(1.24310706121289,0.796739207590962,131.580777111131));
#45284=CARTESIAN_POINT('Ctrl Pts',(0.730392955695213,1.28321263273343,131.607702814841));
#45285=CARTESIAN_POINT('Ctrl Pts',(0.0503226124284044,1.47566126371214,
131.634628518552));
#45286=CARTESIAN_POINT('Ctrl Pts',(-0.64127824057781,1.32998900322893,131.661554222262));
#45287=CARTESIAN_POINT('Ctrl Pts',(-1.1859418690934,0.879573995570998,131.688479925972));
#45288=CARTESIAN_POINT('Ctrl Pts',(-1.45886852662799,0.227620633007125,
131.715405629683));
#45289=CARTESIAN_POINT('Ctrl Pts',(-1.39752204243741,-0.476487850274313,
131.742331333393));
#45290=CARTESIAN_POINT('Ctrl Pts',(-1.01595884561736,-1.07141782445958,
131.769257037104));
#45291=CARTESIAN_POINT('Ctrl Pts',(-0.401607190489387,-1.4208519258194,
131.796182740814));
#45292=CARTESIAN_POINT('Ctrl Pts',(0.304765434899777,-1.44472369685233,
131.823108444524));
#45293=CARTESIAN_POINT('Ctrl Pts',(0.941306613825954,-1.13756335617889,
131.850034148235));
#45294=CARTESIAN_POINT('Ctrl Pts',(1.36216453316536,-0.569751099283571,
131.876959851945));
#45295=CARTESIAN_POINT('Ctrl Pts',(1.47090726889573,0.128609240927045,131.903885555655));
#45296=CARTESIAN_POINT('Ctrl Pts',(1.24261840445668,0.797501116890374,131.930811259366));
#45297=CARTESIAN_POINT('Ctrl Pts',(0.729606173620613,1.28366014270317,131.957736963076));
#45298=CARTESIAN_POINT('Ctrl Pts',(0.0494179817900777,1.47569183560471,
131.984662666786));
#45299=CARTESIAN_POINT('Ctrl Pts',(-0.642093440175745,1.32959563207517,
132.011588370497));
#45300=CARTESIAN_POINT('Ctrl Pts',(-1.18648084958774,0.878846815209795,
132.038514074207));
#45301=CARTESIAN_POINT('Ctrl Pts',(-1.45900779054075,0.226726263649683,
132.065439777918));
#45302=CARTESIAN_POINT('Ctrl Pts',(-1.39722968026521,-0.477344480185226,
132.092365481628));
#45303=CARTESIAN_POINT('Ctrl Pts',(-1.01530184710615,-1.07204043344031,
132.119291185338));
#45304=CARTESIAN_POINT('Ctrl Pts',(-0.400736096042175,-1.42109785445693,
132.146216889049));
#45305=CARTESIAN_POINT('Ctrl Pts',(0.305651028941402,-1.44453659354527,
132.173142592759));
#45306=CARTESIAN_POINT('Ctrl Pts',(0.942003784894263,-1.1369860930341,132.200068296469));
#45307=CARTESIAN_POINT('Ctrl Pts',(1.36251353445943,-0.568915938749493,
132.22699400018));
#45308=CARTESIAN_POINT('Ctrl Pts',(1.47082811283404,0.129510931795882,132.25391970389));
#45309=CARTESIAN_POINT('Ctrl Pts',(1.24212922149168,0.798262763362323,132.2808454076));
#45310=CARTESIAN_POINT('Ctrl Pts',(0.728818964570724,1.28410719647692,132.307771111311));
#45311=CARTESIAN_POINT('Ctrl Pts',(0.0485131144820429,1.47572200663644,
132.334696815021));
#45312=CARTESIAN_POINT('Ctrl Pts',(-0.642909006629927,1.32920183546066,
132.361622518731));
#45313=CARTESIAN_POINT('Ctrl Pts',(-1.18702017535352,0.87811995404865,132.388548222442));
#45314=CARTESIAN_POINT('Ctrl Pts',(-1.45914894676379,0.22583196354202,132.415473926152));
#45315=CARTESIAN_POINT('Ctrl Pts',(-1.39693960210031,-0.478198145289243,
132.442399629863));
#45316=CARTESIAN_POINT('Ctrl Pts',(-1.0146543563804,-1.07266268974653,132.469325333573));
#45317=CARTESIAN_POINT('Ctrl Pts',(-0.39987450728714,-1.42133111811274,
132.496251037283));
#45318=CARTESIAN_POINT('Ctrl Pts',(0.306495977144071,-1.44435231757185,
132.523176740994));
#45319=CARTESIAN_POINT('Ctrl Pts',(0.942669397454339,-1.13635458623572,
132.550102444704));
#45320=CARTESIAN_POINT('Ctrl Pts',(1.22268078144798,-0.757527087161765,
132.568052913844));
#45321=CARTESIAN_POINT('Ctrl Pts',(1.31070900977112,-0.546341674518714,
132.577028148414));
#45322=CARTESIAN_POINT('Ctrl Pts',(-0.644068464422466,1.33997277538071,
131.));
#45323=CARTESIAN_POINT('Ctrl Pts',(-0.859968943773443,1.23619851014301,
131.00897523457));
#45324=CARTESIAN_POINT('Ctrl Pts',(-1.24046603018512,0.922385864810007,
131.02692570371));
#45325=CARTESIAN_POINT('Ctrl Pts',(-1.52710994109882,0.240143529891734,
131.053851407421));
#45326=CARTESIAN_POINT('Ctrl Pts',(-1.46377096569892,-0.497087010650998,
131.080777111131));
#45327=CARTESIAN_POINT('Ctrl Pts',(-1.0650597239944,-1.12045534240007,131.107702814842));
#45328=CARTESIAN_POINT('Ctrl Pts',(-0.422294045014812,-1.48708563881725,
131.134628518552));
#45329=CARTESIAN_POINT('Ctrl Pts',(0.317227981648397,-1.51298531544935,
131.161554222262));
#45330=CARTESIAN_POINT('Ctrl Pts',(0.984066261457807,-1.19221104447402,
131.188479925973));
#45331=CARTESIAN_POINT('Ctrl Pts',(1.42542281590713,-0.598265109305461,
131.215405629683));
#45332=CARTESIAN_POINT('Ctrl Pts',(1.54017040244428,0.132762483030811,131.242331333393));
#45333=CARTESIAN_POINT('Ctrl Pts',(1.30201584504227,0.833369569997161,131.269257037104));
#45334=CARTESIAN_POINT('Ctrl Pts',(0.765528231107528,1.34302520522144,131.296182740814));
#45335=CARTESIAN_POINT('Ctrl Pts',(0.0536337437577054,1.54495099290438,
131.323108444524));
#45336=CARTESIAN_POINT('Ctrl Pts',(-0.670549905646045,1.39287940488435,
131.350034148235));
#45337=CARTESIAN_POINT('Ctrl Pts',(-1.24108926619491,0.921654858529432,
131.376959851945));
#45338=CARTESIAN_POINT('Ctrl Pts',(-1.5272556271745,0.23924989175532,131.403885555655));
#45339=CARTESIAN_POINT('Ctrl Pts',(-1.46347918893899,-0.497974833581676,
131.430811259366));
#45340=CARTESIAN_POINT('Ctrl Pts',(-1.064373158062,-1.12109769997607,131.457736963076));
#45341=CARTESIAN_POINT('Ctrl Pts',(-0.421385411338104,-1.48734145648005,
131.484662666786));
#45342=CARTESIAN_POINT('Ctrl Pts',(0.318155124966732,-1.51278801844595,
131.511588370497));
#45343=CARTESIAN_POINT('Ctrl Pts',(0.984796211311188,-1.19160676986845,
131.538514074207));
#45344=CARTESIAN_POINT('Ctrl Pts',(1.42578918929164,-0.597390541595174,
131.565439777918));
#45345=CARTESIAN_POINT('Ctrl Pts',(1.54008855298824,0.133706844523454,131.592365481628));
#45346=CARTESIAN_POINT('Ctrl Pts',(1.30150468580068,0.834167743387289,131.619291185338));
#45347=CARTESIAN_POINT('Ctrl Pts',(0.764704733786668,1.34349430269641,131.646216889049));
#45348=CARTESIAN_POINT('Ctrl Pts',(0.0526866252480262,1.54498362152493,
131.673142592759));
#45349=CARTESIAN_POINT('Ctrl Pts',(-0.671403663494357,1.39246809367885,
131.700068296469));
#45350=CARTESIAN_POINT('Ctrl Pts',(-1.24165403598166,0.920893873474695,
131.72699400018));
#45351=CARTESIAN_POINT('Ctrl Pts',(-1.52740200954285,0.238313601207157,
131.75391970389));
#45352=CARTESIAN_POINT('Ctrl Pts',(-1.46317364247562,-0.498871890610963,
131.7808454076));
#45353=CARTESIAN_POINT('Ctrl Pts',(-1.06368569482785,-1.1217499783357,131.807771111311));
#45354=CARTESIAN_POINT('Ctrl Pts',(-0.420473550977336,-1.4875994972457,
131.834696815021));
#45355=CARTESIAN_POINT('Ctrl Pts',(0.319082445887751,-1.51259269600317,
131.861622518732));
#45356=CARTESIAN_POINT('Ctrl Pts',(0.985526514083445,-1.19100283849842,
131.888548222442));
#45357=CARTESIAN_POINT('Ctrl Pts',(1.42615513825209,-0.596516381086395,
131.915473926152));
#45358=CARTESIAN_POINT('Ctrl Pts',(1.5400062975897,0.134650936292246,131.942399629863));
#45359=CARTESIAN_POINT('Ctrl Pts',(1.30099307334363,0.834965445012741,131.969325333573));
#45360=CARTESIAN_POINT('Ctrl Pts',(0.763880990933983,1.34396283540829,131.996251037283));
#45361=CARTESIAN_POINT('Ctrl Pts',(0.0517394976421782,1.54501562959783,
132.023176740994));
#45362=CARTESIAN_POINT('Ctrl Pts',(-0.672257158844581,1.39205624307012,
132.050102444704));
#45363=CARTESIAN_POINT('Ctrl Pts',(-1.24221833624253,0.920132532253928,
132.077028148414));
#45364=CARTESIAN_POINT('Ctrl Pts',(-1.52754781567707,0.237377216927905,
132.103953852125));
#45365=CARTESIAN_POINT('Ctrl Pts',(-1.46286754596235,-0.499768762552115,
132.130879555835));
#45366=CARTESIAN_POINT('Ctrl Pts',(-1.06299783240024,-1.12240183571076,
132.157805259545));
#45367=CARTESIAN_POINT('Ctrl Pts',(-0.41956153499722,-1.48785697890927,
132.184730963256));
#45368=CARTESIAN_POINT('Ctrl Pts',(0.320009642611874,-1.51239680311634,
132.211656666966));
#45369=CARTESIAN_POINT('Ctrl Pts',(0.986256436260319,-1.19039845717735,
132.238582370677));
#45370=CARTESIAN_POINT('Ctrl Pts',(1.42652053463166,-0.595641987092175,
132.265508074387));
#45371=CARTESIAN_POINT('Ctrl Pts',(1.53992342300198,0.135594986026619,132.292433778097));
#45372=CARTESIAN_POINT('Ctrl Pts',(1.30048090995801,0.835762871463845,132.319359481808));
#45373=CARTESIAN_POINT('Ctrl Pts',(0.763056801047929,1.34443089049341,132.346285185518));
#45374=CARTESIAN_POINT('Ctrl Pts',(0.0507921222485523,1.54504721797859,
132.373210889228));
#45375=CARTESIAN_POINT('Ctrl Pts',(-0.673111038284911,1.39164394701371,
132.400136592939));
#45376=CARTESIAN_POINT('Ctrl Pts',(-1.24278299799471,0.919371525228328,
132.427062296649));
#45377=CARTESIAN_POINT('Ctrl Pts',(-1.52769560301691,0.23644090515159,132.453988000359));
#45378=CARTESIAN_POINT('Ctrl Pts',(-1.46256384075252,-0.5006625304082,132.48091370407));
#45379=CARTESIAN_POINT('Ctrl Pts',(-1.06231992440674,-1.12305332384367,
132.50783940778));
#45380=CARTESIAN_POINT('Ctrl Pts',(-0.41865947125959,-1.4881012006264,132.53476511149));
#45381=CARTESIAN_POINT('Ctrl Pts',(0.320894284071444,-1.51220387038322,
132.561690815201));
#45382=CARTESIAN_POINT('Ctrl Pts',(0.986953317400244,-1.18973728399054,
132.588616518911));
#45383=CARTESIAN_POINT('Ctrl Pts',(1.28011883766499,-0.793113549367196,
132.606566988051));
#45384=CARTESIAN_POINT('Ctrl Pts',(1.37228238111194,-0.572007248306124,
132.615542222622));
#45385=CARTESIAN_POINT('',(-1.16302251498203,-0.926096109379588,132.5));
#45386=CARTESIAN_POINT('Ctrl Pts',(-1.16302251498205,-0.926096109379563,
132.5));
#45387=CARTESIAN_POINT('Ctrl Pts',(-1.12343887327884,-0.969761157109709,
132.5));
#45388=CARTESIAN_POINT('Ctrl Pts',(-1.08135544679353,-1.01098477954329,
132.5));
#45389=CARTESIAN_POINT('Ctrl Pts',(-1.03694177510552,-1.0495028422266,132.5));
#45390=CARTESIAN_POINT('Ctrl Pts',(-1.02884469989658,-1.05652508647247,
132.5));
#45391=CARTESIAN_POINT('Ctrl Pts',(-1.02067008828795,-1.06345729579591,
132.5));
#45392=CARTESIAN_POINT('Ctrl Pts',(-1.012418858982,-1.07029771551359,132.5));
#45393=CARTESIAN_POINT('Ctrl Pts',(-0.98167242007177,-1.0957870746347,132.5));
#45394=CARTESIAN_POINT('Ctrl Pts',(-0.94986244225381,-1.12000269225618,
132.5));
#45395=CARTESIAN_POINT('Ctrl Pts',(-0.91707717529942,-1.14289362846388,
132.5));
#45396=CARTESIAN_POINT('Ctrl Pts',(-0.901607681935602,-1.15369455274029,
132.5));
#45397=CARTESIAN_POINT('Ctrl Pts',(-0.885920995232433,-1.16420041056655,
132.5));
#45398=CARTESIAN_POINT('Ctrl Pts',(-0.870026136517583,-1.1744050442284,
132.5));
#45399=CARTESIAN_POINT('Ctrl Pts',(-0.859196579215699,-1.18135771156369,
132.5));
#45400=CARTESIAN_POINT('Ctrl Pts',(-0.848277795189246,-1.18816574517481,
132.5));
#45401=CARTESIAN_POINT('Ctrl Pts',(-0.837276000207708,-1.19482592504528,
132.5));
#45402=CARTESIAN_POINT('Ctrl Pts',(-0.7873206039329,-1.22506752882437,132.5));
#45403=CARTESIAN_POINT('Ctrl Pts',(-0.735635042660107,-1.25227756773128,
132.5));
#45404=CARTESIAN_POINT('Ctrl Pts',(-0.682504096094913,-1.27630821846757,
132.5));
#45405=CARTESIAN_POINT('Ctrl Pts',(-0.656532974943956,-1.28805472369579,
132.5));
#45406=CARTESIAN_POINT('Ctrl Pts',(-0.630216202837425,-1.29904081955767,
132.5));
#45407=CARTESIAN_POINT('Ctrl Pts',(-0.603585928569541,-1.30924482499605,
132.5));
#45408=CARTESIAN_POINT('Ctrl Pts',(-0.581793012479383,-1.31759528477973,
132.5));
#45409=CARTESIAN_POINT('Ctrl Pts',(-0.559790126733421,-1.32542192801966,
132.5));
#45410=CARTESIAN_POINT('Ctrl Pts',(-0.537594787919088,-1.33271132314286,
132.5));
#45411=CARTESIAN_POINT('Ctrl Pts',(-0.526294525446042,-1.33642255633695,
132.5));
#45412=CARTESIAN_POINT('Ctrl Pts',(-0.514943176335056,-1.33999474630347,
132.5));
#45413=CARTESIAN_POINT('Ctrl Pts',(-0.503559980499219,-1.34342124510912,
132.5));
#45414=CARTESIAN_POINT('Ctrl Pts',(-0.46487623766045,-1.35506558476089,
132.5));
#45415=CARTESIAN_POINT('Ctrl Pts',(-0.425780872220429,-1.36504338933051,
132.5));
#45416=CARTESIAN_POINT('Ctrl Pts',(-0.386368127474387,-1.37330780015286,
132.5));
#45417=CARTESIAN_POINT('Ctrl Pts',(-0.330299401943935,-1.38506478346002,
132.5));
#45418=CARTESIAN_POINT('Ctrl Pts',(-0.273587986529516,-1.39335645759698,
132.5));
#45419=CARTESIAN_POINT('Ctrl Pts',(-0.216553461875847,-1.39819529077566,
132.5));
#45420=CARTESIAN_POINT('Ctrl Pts',(-0.174416968678751,-1.40177016866855,
132.5));
#45421=CARTESIAN_POINT('Ctrl Pts',(-0.132103871869953,-1.40345934657106,
132.5));
#45422=CARTESIAN_POINT('Ctrl Pts',(-0.0897455132278829,-1.40324976814038,
132.5));
#45423=CARTESIAN_POINT('Ctrl Pts',(-0.0705591202545961,-1.40315483872719,
132.5));
#45424=CARTESIAN_POINT('Ctrl Pts',(-0.0513634969174188,-1.40267014032031,
132.5));
#45425=CARTESIAN_POINT('Ctrl Pts',(-0.0321712203893606,-1.40179344447432,
132.5));
#45426=CARTESIAN_POINT('Ctrl Pts',(-0.0192679054651587,-1.4012040259873,
132.5));
#45427=CARTESIAN_POINT('Ctrl Pts',(-0.00636610869756403,-1.40043740709029,
132.5));
#45428=CARTESIAN_POINT('Ctrl Pts',(0.00653026688444481,-1.39949275165764,
132.5));
#45429=CARTESIAN_POINT('Ctrl Pts',(0.017391646899733,-1.39869715900665,
132.5));
#45430=CARTESIAN_POINT('Ctrl Pts',(0.0282504431870717,-1.39777505085674,
132.5));
#45431=CARTESIAN_POINT('Ctrl Pts',(0.039086617545718,-1.39672789082918,
132.5));
#45432=CARTESIAN_POINT('Ctrl Pts',(0.0949958078773393,-1.3913250736217,
132.5));
#45433=CARTESIAN_POINT('Ctrl Pts',(0.150411388764911,-1.38259070029328,
132.5));
#45434=CARTESIAN_POINT('Ctrl Pts',(0.205031962417632,-1.3705335380372,132.5));
#45435=CARTESIAN_POINT('Ctrl Pts',(0.232388170204765,-1.36449482013398,
132.5));
#45436=CARTESIAN_POINT('Ctrl Pts',(0.259544834917365,-1.3576218081049,132.5));
#45437=CARTESIAN_POINT('Ctrl Pts',(0.286462690387675,-1.34991087227367,
132.5));
#45438=CARTESIAN_POINT('Ctrl Pts',(0.339060168306143,-1.3348437070026,132.5));
#45439=CARTESIAN_POINT('Ctrl Pts',(0.390747678696571,-1.31657948059088,
132.5));
#45440=CARTESIAN_POINT('Ctrl Pts',(0.44125190511673,-1.29524246473403,132.5));
#45441=CARTESIAN_POINT('Ctrl Pts',(0.461191169585947,-1.28681852811902,
132.5));
#45442=CARTESIAN_POINT('Ctrl Pts',(0.480945683432762,-1.2779152214623,132.5));
#45443=CARTESIAN_POINT('Ctrl Pts',(0.50049723434429,-1.26853868323638,132.5));
#45444=CARTESIAN_POINT('Ctrl Pts',(0.51016987966283,-1.26389987330333,132.5));
#45445=CARTESIAN_POINT('Ctrl Pts',(0.519792835446406,-1.25914522637774,
132.5));
#45446=CARTESIAN_POINT('Ctrl Pts',(0.529363810934624,-1.25427541756582,
132.5));
#45447=CARTESIAN_POINT('Ctrl Pts',(0.538615327196273,-1.24956815282879,
132.5));
#45448=CARTESIAN_POINT('Ctrl Pts',(0.54781100101367,-1.24475694311704,132.5));
#45449=CARTESIAN_POINT('Ctrl Pts',(0.556944545350045,-1.23984536162613,
132.5));
#45450=CARTESIAN_POINT('Ctrl Pts',(0.605505112344534,-1.21373182089604,
132.5));
#45451=CARTESIAN_POINT('Ctrl Pts',(0.652353503329041,-1.18476332689692,
132.5));
#45452=CARTESIAN_POINT('Ctrl Pts',(0.697227106842703,-1.1530956883318,132.5));
#45453=CARTESIAN_POINT('Ctrl Pts',(0.741542679959258,-1.12182185600332,
132.5));
#45454=CARTESIAN_POINT('Ctrl Pts',(0.78393305031491,-1.0879149147509,132.5));
#45455=CARTESIAN_POINT('Ctrl Pts',(0.824110992015511,-1.05148810793158,
132.5));
#45456=CARTESIAN_POINT('Ctrl Pts',(0.83326922342897,-1.04318491686743,132.5));
#45457=CARTESIAN_POINT('Ctrl Pts',(0.842312333357698,-1.03475067051344,
132.5));
#45458=CARTESIAN_POINT('Ctrl Pts',(0.851236602531774,-1.02618649277957,
132.5));
#45459=CARTESIAN_POINT('Ctrl Pts',(0.870313615897425,-1.00787923087299,
132.5));
#45460=CARTESIAN_POINT('Ctrl Pts',(0.888847746986408,-0.988978296120459,
132.5));
#45461=CARTESIAN_POINT('Ctrl Pts',(0.906815286248638,-0.969510836032861,
132.5));
#45462=CARTESIAN_POINT('Ctrl Pts',(0.915830068492709,-0.959743504459318,
132.5));
#45463=CARTESIAN_POINT('Ctrl Pts',(0.924702181967323,-0.949833545936108,
132.5));
#45464=CARTESIAN_POINT('Ctrl Pts',(0.933428374226774,-0.939784308310312,
132.5));
#45465=CARTESIAN_POINT('Ctrl Pts',(0.939813745749803,-0.932430801321692,
132.5));
#45466=CARTESIAN_POINT('Ctrl Pts',(0.946120382516669,-0.92500325455595,
132.5));
#45467=CARTESIAN_POINT('Ctrl Pts',(0.952338780021893,-0.917513345854709,
132.5));
#45468=CARTESIAN_POINT('Ctrl Pts',(0.986818201658188,-0.875983720270228,
132.5));
#45469=CARTESIAN_POINT('Ctrl Pts',(1.01865914174794,-0.832458627176748,
132.5));
#45470=CARTESIAN_POINT('Ctrl Pts',(1.04771225996938,-0.787203227418373,
132.5));
#45471=CARTESIAN_POINT('Ctrl Pts',(1.07693733284606,-0.74167997769622,132.5));
#45472=CARTESIAN_POINT('Ctrl Pts',(1.10334204163176,-0.694404893510236,
132.5));
#45473=CARTESIAN_POINT('Ctrl Pts',(1.12672619137727,-0.645625392877356,
132.5));
#45474=CARTESIAN_POINT('Ctrl Pts',(1.15011034112277,-0.596845892244476,
132.5));
#45475=CARTESIAN_POINT('Ctrl Pts',(1.17047445367726,-0.546560987753008,
132.5));
#45476=CARTESIAN_POINT('Ctrl Pts',(1.18756226708949,-0.495010526943894,
132.5));
#45477=CARTESIAN_POINT('Ctrl Pts',(-1.48668131839924,3.04819389219259E-5,
132.46254146791));
#45478=CARTESIAN_POINT('Ctrl Pts',(-1.48655520767872,-0.16343428003251,
132.46866554663));
#45479=CARTESIAN_POINT('Ctrl Pts',(-1.45963517263437,-0.326939632586996,
132.47478962535));
#45480=CARTESIAN_POINT('Ctrl Pts',(-1.40671181507228,-0.481543756720818,
132.48091370407));
#45481=CARTESIAN_POINT('Ctrl Pts',(-1.35173152550569,-0.642156762104989,
132.487275802713));
#45482=CARTESIAN_POINT('Ctrl Pts',(-1.26868733036522,-0.793163178418914,
132.493637901357));
#45483=CARTESIAN_POINT('Ctrl Pts',(-1.16302251498203,-0.926096109379588,
132.5));
#45484=CARTESIAN_POINT('',(-0.746857044344933,-1.04763739686609,131.));
#45485=CARTESIAN_POINT('Ctrl Pts',(-0.746861959042824,-1.04760678153428,
131.));
#45486=CARTESIAN_POINT('Ctrl Pts',(-0.79290540902848,-1.01977850456588,
131.));
#45487=CARTESIAN_POINT('Ctrl Pts',(-0.837111201294298,-0.989131878238612,
131.));
#45488=CARTESIAN_POINT('Ctrl Pts',(-0.879206377167662,-0.955837561748656,
131.));
#45489=CARTESIAN_POINT('Ctrl Pts',(-0.884791465636455,-0.95142015050743,
131.));
#45490=CARTESIAN_POINT('Ctrl Pts',(-0.890339378075958,-0.946956059295192,
131.));
#45491=CARTESIAN_POINT('Ctrl Pts',(-0.895849453575902,-0.942445622075628,
131.));
#45492=CARTESIAN_POINT('Ctrl Pts',(-0.926217339091838,-0.917587080461831,
131.));
#45493=CARTESIAN_POINT('Ctrl Pts',(-0.955436613451353,-0.891321827243511,
131.));
#45494=CARTESIAN_POINT('Ctrl Pts',(-0.983445198717416,-0.863753973035975,
131.));
#45495=CARTESIAN_POINT('Ctrl Pts',(-0.992679469403162,-0.854665008864478,
131.));
#45496=CARTESIAN_POINT('Ctrl Pts',(-1.00178207011453,-0.845434352437698,
131.));
#45497=CARTESIAN_POINT('Ctrl Pts',(-1.01075055479975,-0.836065450228404,
131.));
#45498=CARTESIAN_POINT('Ctrl Pts',(-1.01912420496792,-0.827317940218179,
131.));
#45499=CARTESIAN_POINT('Ctrl Pts',(-1.02737472791407,-0.818456358266283,
131.));
#45500=CARTESIAN_POINT('Ctrl Pts',(-1.0354984320536,-0.809486419032962,
131.));
#45501=CARTESIAN_POINT('Ctrl Pts',(-1.07199487788031,-0.769188188610594,
131.));
#45502=CARTESIAN_POINT('Ctrl Pts',(-1.10594836061416,-0.726691494335613,
131.));
#45503=CARTESIAN_POINT('Ctrl Pts',(-1.13720585307844,-0.682279068598729,
131.));
#45504=CARTESIAN_POINT('Ctrl Pts',(-1.15346249868424,-0.659180700534707,
131.));
#45505=CARTESIAN_POINT('Ctrl Pts',(-1.16898942799938,-0.635563406373612,
131.));
#45506=CARTESIAN_POINT('Ctrl Pts',(-1.18376147727168,-0.611462797325301,
131.));
#45507=CARTESIAN_POINT('Ctrl Pts',(-1.19227111129058,-0.597579323282302,
131.));
#45508=CARTESIAN_POINT('Ctrl Pts',(-1.20053018904277,-0.583535413960466,
131.));
#45509=CARTESIAN_POINT('Ctrl Pts',(-1.20853345336714,-0.569337528515594,
131.));
#45510=CARTESIAN_POINT('Ctrl Pts',(-1.21501758519943,-0.557834602055454,
131.));
#45511=CARTESIAN_POINT('Ctrl Pts',(-1.2213347587292,-0.546228423437439,
131.));
#45512=CARTESIAN_POINT('Ctrl Pts',(-1.22747166438142,-0.534543038687395,
131.));
#45513=CARTESIAN_POINT('Ctrl Pts',(-1.24489028000614,-0.50137596118562,
131.));
#45514=CARTESIAN_POINT('Ctrl Pts',(-1.2608770606582,-0.46753740688374,131.));
#45515=CARTESIAN_POINT('Ctrl Pts',(-1.27538574703159,-0.43311685629096,
131.));
#45516=CARTESIAN_POINT('Ctrl Pts',(-1.29685816110231,-0.382175489453921,
131.));
#45517=CARTESIAN_POINT('Ctrl Pts',(-1.31509556112442,-0.329960528095882,
131.));
#45518=CARTESIAN_POINT('Ctrl Pts',(-1.33010366412696,-0.276796734514434,
131.));
#45519=CARTESIAN_POINT('Ctrl Pts',(-1.34135974137886,-0.236923889328347,
131.));
#45520=CARTESIAN_POINT('Ctrl Pts',(-1.35079846340778,-0.196516449979369,
131.));
#45521=CARTESIAN_POINT('Ctrl Pts',(-1.35840472687476,-0.155702664587729,
131.));
#45522=CARTESIAN_POINT('Ctrl Pts',(-1.36226900717259,-0.134967660146506,
131.));
#45523=CARTESIAN_POINT('Ctrl Pts',(-1.36566007611252,-0.114127685083141,
131.));
#45524=CARTESIAN_POINT('Ctrl Pts',(-1.36857437917471,-0.0931991623570564,
131.));
#45525=CARTESIAN_POINT('Ctrl Pts',(-1.37032032486804,-0.0806609796967288,
131.));
#45526=CARTESIAN_POINT('Ctrl Pts',(-1.37189513129338,-0.0680910121185238,
131.));
#45527=CARTESIAN_POINT('Ctrl Pts',(-1.37329784488209,-0.0554927709829172,
131.));
#45528=CARTESIAN_POINT('Ctrl Pts',(-1.37435287170058,-0.0460172213261885,
131.));
#45529=CARTESIAN_POINT('Ctrl Pts',(-1.37530946257138,-0.0365353663362607,
131.));
#45530=CARTESIAN_POINT('Ctrl Pts',(-1.37616775261068,-0.0270488533894786,
131.));
#45531=CARTESIAN_POINT('Ctrl Pts',(-1.38126770774191,0.0293199592087556,
131.));
#45532=CARTESIAN_POINT('Ctrl Pts',(-1.38290082952566,0.0858515591714624,
131.));
#45533=CARTESIAN_POINT('Ctrl Pts',(-1.3810680521945,0.142217815274853,131.));
#45534=CARTESIAN_POINT('Ctrl Pts',(-1.38026175318832,0.167015184549204,
131.));
#45535=CARTESIAN_POINT('Ctrl Pts',(-1.3787840345135,0.191780836376777,131.));
#45536=CARTESIAN_POINT('Ctrl Pts',(-1.37663194421336,0.216487800262018,
131.));
#45537=CARTESIAN_POINT('Ctrl Pts',(-1.37167800010617,0.273361305122912,
131.));
#45538=CARTESIAN_POINT('Ctrl Pts',(-1.3631544857951,0.329924039407384,131.));
#45539=CARTESIAN_POINT('Ctrl Pts',(-1.35119091111081,0.385880739631646,
131.));
#45540=CARTESIAN_POINT('Ctrl Pts',(-1.34632600887317,0.408635132304057,
131.));
#45541=CARTESIAN_POINT('Ctrl Pts',(-1.34089162405852,0.431289287179278,
131.));
#45542=CARTESIAN_POINT('Ctrl Pts',(-1.33489389522501,0.45382298681954,131.));
#45543=CARTESIAN_POINT('Ctrl Pts',(-1.33224239577941,0.463784772982573,
131.));
#45544=CARTESIAN_POINT('Ctrl Pts',(-1.32948021180854,0.473724958560968,
131.));
#45545=CARTESIAN_POINT('Ctrl Pts',(-1.32660959425527,0.483635551674743,
131.));
#45546=CARTESIAN_POINT('Ctrl Pts',(-1.31067425301938,0.538651129399031,
131.));
#45547=CARTESIAN_POINT('Ctrl Pts',(-1.29146044376945,0.592556875483699,
131.));
#45548=CARTESIAN_POINT('Ctrl Pts',(-1.26913667157012,0.645068264124258,
131.));
#45549=CARTESIAN_POINT('Ctrl Pts',(-1.24656696606482,0.698158152639027,
131.));
#45550=CARTESIAN_POINT('Ctrl Pts',(-1.2208182026231,0.7498238393096,131.));
#45551=CARTESIAN_POINT('Ctrl Pts',(-1.19201211730027,0.799766583668426,
131.));
#45552=CARTESIAN_POINT('Ctrl Pts',(-1.18039996771779,0.819899226183185,
131.));
#45553=CARTESIAN_POINT('Ctrl Pts',(-1.16829042624204,0.839751747079717,
131.));
#45554=CARTESIAN_POINT('Ctrl Pts',(-1.1556892086837,0.859303760062855,131.));
#45555=CARTESIAN_POINT('Ctrl Pts',(-1.13970882525568,0.884098877107183,
131.));
#45556=CARTESIAN_POINT('Ctrl Pts',(-1.12293779488653,0.908410786623963,
131.));
#45557=CARTESIAN_POINT('Ctrl Pts',(-1.10540618886941,0.93221250033084,131.));
#45558=CARTESIAN_POINT('Ctrl Pts',(-1.09666464487149,0.944080422036999,
131.));
#45559=CARTESIAN_POINT('Ctrl Pts',(-1.08773396101947,0.955821468651418,
131.));
#45560=CARTESIAN_POINT('Ctrl Pts',(-1.07861760001237,0.96743209119293,131.));
#45561=CARTESIAN_POINT('Ctrl Pts',(-1.07225241782588,0.97553880479475,131.));
#45562=CARTESIAN_POINT('Ctrl Pts',(-1.06579920898365,0.98357864484497,131.));
#45563=CARTESIAN_POINT('Ctrl Pts',(-1.05926555171675,0.991543240500075,
131.));
#45564=CARTESIAN_POINT('Ctrl Pts',(-1.02223281978106,1.03668652301743,131.));
#45565=CARTESIAN_POINT('Ctrl Pts',(-0.982563863156014,1.07948549390314,
131.));
#45566=CARTESIAN_POINT('Ctrl Pts',(-0.940543142400786,1.11976824348413,
131.));
#45567=CARTESIAN_POINT('Ctrl Pts',(-0.896036753133427,1.16243385467282,
131.));
#45568=CARTESIAN_POINT('Ctrl Pts',(-0.848891793255228,1.20227795490809,
131.));
#45569=CARTESIAN_POINT('Ctrl Pts',(-0.799392172671262,1.23906470001876,
131.));
#45570=CARTESIAN_POINT('Ctrl Pts',(-0.752607904601772,1.27383347045292,
131.));
#45571=CARTESIAN_POINT('Ctrl Pts',(-0.703719130108104,1.30587158459506,
131.));
#45572=CARTESIAN_POINT('Ctrl Pts',(-0.652930875785528,1.33494126253536,
131.));
#45573=CARTESIAN_POINT('Ctrl Pts',(-0.649983132457026,1.33662846266368,
131.));
#45574=CARTESIAN_POINT('Ctrl Pts',(-0.647028982870071,1.33830565070331,
131.));
#45575=CARTESIAN_POINT('Ctrl Pts',(-0.644068464422466,1.33997277538071,
131.));
#45576=CARTESIAN_POINT('Ctrl Pts',(-0.746861959043068,-1.04760678153411,
131.));
#45577=CARTESIAN_POINT('Ctrl Pts',(-0.627129610382755,-1.13281069019958,
131.006362098643));
#45578=CARTESIAN_POINT('Ctrl Pts',(-0.303340278729474,-1.28908730893346,
131.021699431857));
#45579=CARTESIAN_POINT('Ctrl Pts',(0.274526574308514,-1.30932546829921,
131.046011999641));
#45580=CARTESIAN_POINT('Ctrl Pts',(0.851603122293372,-1.03172996338952,
131.072937703351));
#45581=CARTESIAN_POINT('Ctrl Pts',(1.23354957705434,-0.517733871181562,
131.099863407061));
#45582=CARTESIAN_POINT('Ctrl Pts',(1.3328512265448,0.114891597751729,131.126789110772));
#45583=CARTESIAN_POINT('Ctrl Pts',(1.12675416518279,0.721191403089574,131.153714814482));
#45584=CARTESIAN_POINT('Ctrl Pts',(0.662482047549443,1.16224333958056,131.180640518192));
#45585=CARTESIAN_POINT('Ctrl Pts',(0.0464142156206867,1.33698831153762,
131.207566221903));
#45586=CARTESIAN_POINT('Ctrl Pts',(-0.580288559487598,1.20538676777764,
131.234491925613));
#45587=CARTESIAN_POINT('Ctrl Pts',(-1.07402878803166,0.797592790182427,
131.261417629323));
#45588=CARTESIAN_POINT('Ctrl Pts',(-1.26566344030531,0.340612318858289,
131.282253402549));
#45589=CARTESIAN_POINT('Ctrl Pts',(-1.28660881016683,0.0666735963628725,
131.294113941204));
#45590=CARTESIAN_POINT('Ctrl Pts',(-1.28655804524971,2.50455016348322E-5,
131.296999245288));
#45591=CARTESIAN_POINT('Origin',(0.,0.,130.353000754712));
#45592=CARTESIAN_POINT('',(0.746857044345347,-1.04763739686579,131.));
#45593=CARTESIAN_POINT('Origin',(0.,0.,131.));
#45594=CARTESIAN_POINT('Ctrl Pts',(0.746857044345091,-1.04763739686597,
131.));
#45595=CARTESIAN_POINT('Ctrl Pts',(0.915655560497863,-0.927301523747248,
131.00897523457));
#45596=CARTESIAN_POINT('Ctrl Pts',(1.19383071914578,-0.603582305382327,
131.02692570371));
#45597=CARTESIAN_POINT('Ctrl Pts',(1.33763256702269,0.0204649803060436,
131.053851407421));
#45598=CARTESIAN_POINT('Ctrl Pts',(1.17488299294373,0.639781288322262,131.080777111131));
#45599=CARTESIAN_POINT('Ctrl Pts',(0.742945664266514,1.11253782599317,131.107702814841));
#45600=CARTESIAN_POINT('Ctrl Pts',(0.140763636876506,1.33036910873258,131.134628518552));
#45601=CARTESIAN_POINT('Ctrl Pts',(-0.49366903146045,1.24337802076997,131.161554222262));
#45602=CARTESIAN_POINT('Ctrl Pts',(-1.01498908290289,0.871488239228939,
131.188479925973));
#45603=CARTESIAN_POINT('Ctrl Pts',(-1.2525149888957,0.401316727103227,131.210628770122));
#45604=CARTESIAN_POINT('Ctrl Pts',(-1.28652850751777,0.0969951814981651,
131.223802379702));
#45605=CARTESIAN_POINT('Ctrl Pts',(-1.28651324097226,5.80358258382013E-6,
131.228000754712));
#45606=CARTESIAN_POINT('Ctrl Pts',(0.863027389440352,-1.21059280961881,
130.884457777378));
#45607=CARTESIAN_POINT('Ctrl Pts',(1.05808177613958,-1.07153921801113,130.893433011949));
#45608=CARTESIAN_POINT('Ctrl Pts',(1.37952586345563,-0.69746689178419,130.911383481089));
#45609=CARTESIAN_POINT('Ctrl Pts',(1.54569545951096,0.0236482184404665,
130.938309184799));
#45610=CARTESIAN_POINT('Ctrl Pts',(1.35763090135572,0.739296468118232,130.96523488851));
#45611=CARTESIAN_POINT('Ctrl Pts',(0.858507611306259,1.28558821650061,130.99216059222));
#45612=CARTESIAN_POINT('Ctrl Pts',(0.162658804628651,1.53730220206782,131.01908629593));
#45613=CARTESIAN_POINT('Ctrl Pts',(-0.570457089070449,1.43678003103469,
131.046011999641));
#45614=CARTESIAN_POINT('Ctrl Pts',(-1.17286619328369,1.00704442131793,131.072937703351));
#45615=CARTESIAN_POINT('Ctrl Pts',(-1.50653382270734,0.34656482765933,131.099863407061));
#45616=CARTESIAN_POINT('Ctrl Pts',(-1.49500734612767,-0.393324007405797,
131.126789110772));
#45617=CARTESIAN_POINT('Ctrl Pts',(-1.14092708773515,-1.04308939023749,
131.153714814482));
#45618=CARTESIAN_POINT('Ctrl Pts',(-0.525424324038318,-1.45384987150975,
131.180640518192));
#45619=CARTESIAN_POINT('Ctrl Pts',(0.210469861461765,-1.53148704892802,
131.207566221903));
#45620=CARTESIAN_POINT('Ctrl Pts',(0.898138679547195,-1.25821187382816,
131.234491925613));
#45621=CARTESIAN_POINT('Ctrl Pts',(1.38001538427226,-0.696640351025329,
131.261417629323));
#45622=CARTESIAN_POINT('Ctrl Pts',(1.54568670044473,0.0245536163580204,
131.288343333034));
#45623=CARTESIAN_POINT('Ctrl Pts',(1.35719207190964,0.740121575040211,131.315269036744));
#45624=CARTESIAN_POINT('Ctrl Pts',(0.857721606883694,1.28610416068526,131.342194740455));
#45625=CARTESIAN_POINT('Ctrl Pts',(0.16171986348354,1.53739941243649,131.369120444165));
#45626=CARTESIAN_POINT('Ctrl Pts',(-0.571337040454812,1.43642760104845,
131.396046147875));
#45627=CARTESIAN_POINT('Ctrl Pts',(-1.17348247162191,1.00632457743981,131.422971851586));
#45628=CARTESIAN_POINT('Ctrl Pts',(-1.50674577582422,0.345640612600471,
131.449897555296));
#45629=CARTESIAN_POINT('Ctrl Pts',(-1.49476573901151,-0.394240600839361,
131.476823259006));
#45630=CARTESIAN_POINT('Ctrl Pts',(-1.14028736834168,-1.04378876379489,
131.503748962717));
#45631=CARTESIAN_POINT('Ctrl Pts',(-0.52453292370194,-1.45417174974665,
131.530674666427));
#45632=CARTESIAN_POINT('Ctrl Pts',(0.211408683204288,-1.53135777481333,
131.557600370137));
#45633=CARTESIAN_POINT('Ctrl Pts',(0.898909842300872,-1.25766106771139,
131.584526073848));
#45634=CARTESIAN_POINT('Ctrl Pts',(1.38044218951963,-0.695794242015611,
131.611451777558));
#45635=CARTESIAN_POINT('Ctrl Pts',(1.54567136120299,0.0255011565974578,
131.638377481268));
#45636=CARTESIAN_POINT('Ctrl Pts',(1.35673810319962,0.740953429817608,131.665303184979));
#45637=CARTESIAN_POINT('Ctrl Pts',(0.856933029143843,1.28662972505494,131.692228888689));
#45638=CARTESIAN_POINT('Ctrl Pts',(0.160777365112824,1.53749826168993,131.7191545924));
#45639=CARTESIAN_POINT('Ctrl Pts',(-0.572217502707418,1.43607708547494,
131.74608029611));
#45640=CARTESIAN_POINT('Ctrl Pts',(-1.17409915580718,1.00560501100616,131.77300599982));
#45641=CARTESIAN_POINT('Ctrl Pts',(-1.50695737989574,0.344716870779641,
131.799931703531));
#45642=CARTESIAN_POINT('Ctrl Pts',(-1.49452377772872,-0.395156859511377,
131.826857407241));
#45643=CARTESIAN_POINT('Ctrl Pts',(-1.1396472826949,-1.04448759535701,131.853783110951));
#45644=CARTESIAN_POINT('Ctrl Pts',(-0.523641377640934,-1.45449302970016,
131.880708814662));
#45645=CARTESIAN_POINT('Ctrl Pts',(0.212347408168359,-1.53122788771527,
131.907634518372));
#45646=CARTESIAN_POINT('Ctrl Pts',(0.899680654475158,-1.25710977484312,
131.934560222082));
#45647=CARTESIAN_POINT('Ctrl Pts',(1.38086847141359,-0.694947862086922,
131.961485925793));
#45648=CARTESIAN_POINT('Ctrl Pts',(1.54565543818633,0.0264486909784084,
131.988411629503));
#45649=CARTESIAN_POINT('Ctrl Pts',(1.35628362403499,0.74178500846249,132.015337333214));
#45650=CARTESIAN_POINT('Ctrl Pts',(0.856144129802408,1.28715480656056,132.042263036924));
#45651=CARTESIAN_POINT('Ctrl Pts',(0.159834808689029,1.53759653349821,132.069188740634));
#45652=CARTESIAN_POINT('Ctrl Pts',(-0.573097745361402,1.43572602897267,
132.096114444345));
#45653=CARTESIAN_POINT('Ctrl Pts',(-1.17471538828929,1.00488506607529,132.123040148055));
#45654=CARTESIAN_POINT('Ctrl Pts',(-1.50716839969975,0.343792993074946,
132.149965851765));
#45655=CARTESIAN_POINT('Ctrl Pts',(-1.49428121352215,-0.396072971222168,
132.176891555476));
#45656=CARTESIAN_POINT('Ctrl Pts',(-1.13900670115657,-1.04518606185716,
132.203817259186));
#45657=CARTESIAN_POINT('Ctrl Pts',(-0.522749472625893,-1.45481376279687,
132.230742962896));
#45658=CARTESIAN_POINT('Ctrl Pts',(0.2132863055228,-1.53109754478736,132.257668666607));
#45659=CARTESIAN_POINT('Ctrl Pts',(0.900451768791074,-1.25655797749756,
132.284594370317));
#45660=CARTESIAN_POINT('Ctrl Pts',(1.38129516574151,-0.694101749712872,
132.311520074027));
#45661=CARTESIAN_POINT('Ctrl Pts',(1.5456414785732,0.027396491834726,132.338445777738));
#45662=CARTESIAN_POINT('Ctrl Pts',(1.35583202819204,0.742613936399278,132.365371481448));
#45663=CARTESIAN_POINT('Ctrl Pts',(0.855365099195844,1.28768122148057,132.392297185159));
#45664=CARTESIAN_POINT('Ctrl Pts',(0.158904313890113,1.53768343657436,132.419222888869));
#45665=CARTESIAN_POINT('Ctrl Pts',(-0.57393656553719,1.4353851436209,132.446148592579));
#45666=CARTESIAN_POINT('Ctrl Pts',(-1.17528939195008,1.00411479336165,132.47307429629));
#45667=CARTESIAN_POINT('Ctrl Pts',(-1.39656552507781,0.563327679862032,
132.49102476543));
#45668=CARTESIAN_POINT('Ctrl Pts',(-1.44969557651745,0.32974832986801,132.5));
#45669=CARTESIAN_POINT('Ctrl Pts',(0.824303941075265,-1.1562743387012,130.922971851586));
#45670=CARTESIAN_POINT('Ctrl Pts',(1.01060637092568,-1.02345998658984,130.931947086156));
#45671=CARTESIAN_POINT('Ctrl Pts',(1.31762748201901,-0.666172029650235,
130.949897555296));
#45672=CARTESIAN_POINT('Ctrl Pts',(1.47634116201487,0.0225871390623255,
130.976823259006));
#45673=CARTESIAN_POINT('Ctrl Pts',(1.29671493188506,0.706124741519575,131.003748962717));
#45674=CARTESIAN_POINT('Ctrl Pts',(0.81998696229301,1.22790475299813,131.030674666427));
#45675=CARTESIAN_POINT('Ctrl Pts',(0.155360415377937,1.46832450428941,131.057600370137));
#45676=CARTESIAN_POINT('Ctrl Pts',(-0.544861069867116,1.37231269427979,
131.084526073848));
#45677=CARTESIAN_POINT('Ctrl Pts',(-1.12024048982342,0.961859027288264,
131.111451777558));
#45678=CARTESIAN_POINT('Ctrl Pts',(-1.43893668105498,0.331014701008398,
131.138377481268));
#45679=CARTESIAN_POINT('Ctrl Pts',(-1.42792738959148,-0.375675828358543,
131.165303184979));
#45680=CARTESIAN_POINT('Ctrl Pts',(-1.08973447008383,-0.996286683119207,
131.192228888689));
#45681=CARTESIAN_POINT('Ctrl Pts',(-0.501848894184519,-1.3886166226942,
131.2191545924));
#45682=CARTESIAN_POINT('Ctrl Pts',(0.201026222809685,-1.46277027309148,
131.24608029611));
#45683=CARTESIAN_POINT('Ctrl Pts',(0.857839811622868,-1.20175676808682,
131.27300599982));
#45684=CARTESIAN_POINT('Ctrl Pts',(1.31809503837159,-0.665382575209595,
131.299931703531));
#45685=CARTESIAN_POINT('Ctrl Pts',(1.47633279596194,0.0234519123949133,
131.326857407241));
#45686=CARTESIAN_POINT('Ctrl Pts',(1.29629579241592,0.706912826458615,131.353783110951));
#45687=CARTESIAN_POINT('Ctrl Pts',(0.819236225350996,1.22839754712029,131.380708814662));
#45688=CARTESIAN_POINT('Ctrl Pts',(0.154463603879457,1.46841735289536,131.407634518372));
#45689=CARTESIAN_POINT('Ctrl Pts',(-0.545701538435044,1.37197607758584,
131.434560222082));
#45690=CARTESIAN_POINT('Ctrl Pts',(-1.12082911617435,0.961171482312347,
131.461485925793));
#45691=CARTESIAN_POINT('Ctrl Pts',(-1.43913912398055,0.330131954846758,
131.488411629503));
#45692=CARTESIAN_POINT('Ctrl Pts',(-1.42769662322128,-0.376551294871999,
131.515337333214));
#45693=CARTESIAN_POINT('Ctrl Pts',(-1.08912345446176,-0.996954676263693,
131.542263036924));
#45694=CARTESIAN_POINT('Ctrl Pts',(-0.500997490371219,-1.38892405847489,
131.569188740634));
#45695=CARTESIAN_POINT('Ctrl Pts',(0.20192292026309,-1.46264679941786,131.596114444345));
#45696=CARTESIAN_POINT('Ctrl Pts',(0.85857637283152,-1.20123067626358,131.623040148055));
#45697=CARTESIAN_POINT('Ctrl Pts',(1.3185026931596,-0.664574430532121,131.649965851765));
#45698=CARTESIAN_POINT('Ctrl Pts',(1.47631814498149,0.0243569371522413,
131.676891555476));
#45699=CARTESIAN_POINT('Ctrl Pts',(1.29586219297125,0.707707356481415,131.703817259186));
#45700=CARTESIAN_POINT('Ctrl Pts',(0.818483030554682,1.22889952977637,131.730742962896));
#45701=CARTESIAN_POINT('Ctrl Pts',(0.153563394765651,1.46851176685045,131.757668666607));
#45702=CARTESIAN_POINT('Ctrl Pts',(-0.546542494948905,1.37164128940625,
131.784594370317));
#45703=CARTESIAN_POINT('Ctrl Pts',(-1.12141813016224,0.960484202332149,
131.811520074027));
#45704=CARTESIAN_POINT('Ctrl Pts',(-1.43934123352219,0.32924966068928,131.838445777738));
#45705=CARTESIAN_POINT('Ctrl Pts',(-1.42746551857567,-0.377426441644429,
131.865371481448));
#45706=CARTESIAN_POINT('Ctrl Pts',(-1.08851208901992,-0.997622151731854,
131.892297185159));
#45707=CARTESIAN_POINT('Ctrl Pts',(-0.500145947371855,-1.38923092281675,
131.919222888869));
#45708=CARTESIAN_POINT('Ctrl Pts',(0.202819525280424,-1.462522740265,131.946148592579));
#45709=CARTESIAN_POINT('Ctrl Pts',(0.859312599191039,-1.20070411952904,
131.97307429629));
#45710=CARTESIAN_POINT('Ctrl Pts',(1.31890984807669,-0.663766027091625,
132.));
#45711=CARTESIAN_POINT('Ctrl Pts',(1.47630293641969,0.0252619563139483,
132.02692570371));
#45712=CARTESIAN_POINT('Ctrl Pts',(1.29542810597572,0.70850162276158,132.053851407421));
#45713=CARTESIAN_POINT('Ctrl Pts',(0.817729528586826,1.22940105123416,132.080777111131));
#45714=CARTESIAN_POINT('Ctrl Pts',(0.152663130203568,1.46860562926994,132.107702814841));
#45715=CARTESIAN_POINT('Ctrl Pts',(-0.547383241717385,1.371305984569,132.134628518552));
#45716=CARTESIAN_POINT('Ctrl Pts',(-1.12200671271459,0.959796560837642,
132.161554222262));
#45717=CARTESIAN_POINT('Ctrl Pts',(-1.43954278501201,0.328367236744954,
132.188479925973));
#45718=CARTESIAN_POINT('Ctrl Pts',(-1.42723383805905,-0.378301448049683,
132.215405629683));
#45719=CARTESIAN_POINT('Ctrl Pts',(-1.08790024993684,-0.998289278518124,
132.242331333393));
#45720=CARTESIAN_POINT('Ctrl Pts',(-0.499294061524478,-1.38953726483889,
132.269257037104));
#45721=CARTESIAN_POINT('Ctrl Pts',(0.203716294953091,-1.46239824573507,
132.296182740814));
#45722=CARTESIAN_POINT('Ctrl Pts',(0.8600491141353,-1.20017708095276,132.323108444524));
#45723=CARTESIAN_POINT('Ctrl Pts',(1.31931739692212,-0.662957879200776,
132.350034148235));
#45724=CARTESIAN_POINT('Ctrl Pts',(1.47628960316484,0.0261672299944563,
132.376959851945));
#45725=CARTESIAN_POINT('Ctrl Pts',(1.2949967729292,0.709293357269108,132.403885555655));
#45726=CARTESIAN_POINT('Ctrl Pts',(0.816985452550462,1.22990384627695,132.430811259366));
#45727=CARTESIAN_POINT('Ctrl Pts',(0.15177438606951,1.46868863306454,132.457736963076));
#45728=CARTESIAN_POINT('Ctrl Pts',(-0.54818442460592,1.37098039450968,132.484662666787));
#45729=CARTESIAN_POINT('Ctrl Pts',(-1.12255496122393,0.959060849733538,
132.511588370497));
#45730=CARTESIAN_POINT('Ctrl Pts',(-1.33390258568503,0.538051552370983,
132.529538839637));
#45731=CARTESIAN_POINT('Ctrl Pts',(-1.38464872807528,0.314952747964871,
132.538514074207));
#45732=CARTESIAN_POINT('Ctrl Pts',(0.785580492710178,-1.10195586778359,
130.961485925793));
#45733=CARTESIAN_POINT('Ctrl Pts',(0.96313096571177,-0.975380755168544,
130.970461160363));
#45734=CARTESIAN_POINT('Ctrl Pts',(1.2557291005824,-0.634877167516282,130.988411629503));
#45735=CARTESIAN_POINT('Ctrl Pts',(1.40698686451878,0.0215260596841844,
131.015337333214));
#45736=CARTESIAN_POINT('Ctrl Pts',(1.23579896241439,0.672953014920919,131.042263036924));
#45737=CARTESIAN_POINT('Ctrl Pts',(0.781466313279763,1.17022128949565,131.069188740634));
#45738=CARTESIAN_POINT('Ctrl Pts',(0.14806202612722,1.399346806511,131.096114444345));
#45739=CARTESIAN_POINT('Ctrl Pts',(-0.519265050663783,1.30784535752488,
131.123040148055));
#45740=CARTESIAN_POINT('Ctrl Pts',(-1.06761478636316,0.916673633258601,
131.149965851765));
#45741=CARTESIAN_POINT('Ctrl Pts',(-1.37133953940263,0.315464574357466,
131.176891555476));
#45742=CARTESIAN_POINT('Ctrl Pts',(-1.36084743305529,-0.358027649311288,
131.203817259186));
#45743=CARTESIAN_POINT('Ctrl Pts',(-1.0385418524325,-0.949483976000927,
131.230742962896));
#45744=CARTESIAN_POINT('Ctrl Pts',(-0.478273464330721,-1.32338337387865,
131.257668666607));
#45745=CARTESIAN_POINT('Ctrl Pts',(0.191582584157607,-1.39405349725495,
131.284594370317));
#45746=CARTESIAN_POINT('Ctrl Pts',(0.817540943698542,-1.14530166234549,
131.311520074027));
#45747=CARTESIAN_POINT('Ctrl Pts',(1.25617469247093,-0.63412479939386,131.338445777738));
#45748=CARTESIAN_POINT('Ctrl Pts',(1.40697889147916,0.0223502084318068,
131.365371481448));
#45749=CARTESIAN_POINT('Ctrl Pts',(1.23539951292219,0.673704077877018,131.392297185159));
#45750=CARTESIAN_POINT('Ctrl Pts',(0.7807508438183,1.17069093355532,131.419222888869));
#45751=CARTESIAN_POINT('Ctrl Pts',(0.147207344275373,1.39943529335423,131.446148592579));
#45752=CARTESIAN_POINT('Ctrl Pts',(-0.520066036415274,1.30752455412324,
131.47307429629));
#45753=CARTESIAN_POINT('Ctrl Pts',(-1.06817576072678,0.916018387184884,
131.5));
#45754=CARTESIAN_POINT('Ctrl Pts',(-1.37153247213689,0.314623297093045,
131.52692570371));
#45755=CARTESIAN_POINT('Ctrl Pts',(-1.36062750743105,-0.358861988904637,
131.553851407421));
#45756=CARTESIAN_POINT('Ctrl Pts',(-1.03795954058184,-0.950120588732497,
131.580777111131));
#45757=CARTESIAN_POINT('Ctrl Pts',(-0.477462057040497,-1.32367636720312,
131.607702814841));
#45758=CARTESIAN_POINT('Ctrl Pts',(0.19243715732189,-1.39393582402238,131.634628518552));
#45759=CARTESIAN_POINT('Ctrl Pts',(0.81824290336217,-1.14480028481577,131.661554222262));
#45760=CARTESIAN_POINT('Ctrl Pts',(1.25656319679956,-0.633354619048632,
131.688479925973));
#45761=CARTESIAN_POINT('Ctrl Pts',(1.40696492875998,0.0232127177070255,
131.715405629683));
#45762=CARTESIAN_POINT('Ctrl Pts',(1.23498628274288,0.674461283145224,131.742331333393));
#45763=CARTESIAN_POINT('Ctrl Pts',(0.780033031965522,1.17116933449779,131.769257037104));
#45764=CARTESIAN_POINT('Ctrl Pts',(0.146349424418478,1.39952527201097,131.796182740814));
#45765=CARTESIAN_POINT('Ctrl Pts',(-0.520867487190394,1.30720549333756,
131.823108444524));
#45766=CARTESIAN_POINT('Ctrl Pts',(-1.0687371045173,0.91536339365814,131.850034148235));
#45767=CARTESIAN_POINT('Ctrl Pts',(-1.37172508714864,0.313782450598919,
131.876959851945));
#45768=CARTESIAN_POINT('Ctrl Pts',(-1.36040725942262,-0.35969602377748,
131.903885555655));
#45769=CARTESIAN_POINT('Ctrl Pts',(-1.03737689534494,-0.950756708106701,
131.930811259366));
#45770=CARTESIAN_POINT('Ctrl Pts',(-0.476650517102775,-1.32396881593333,
131.957736963076));
#45771=CARTESIAN_POINT('Ctrl Pts',(0.193291642392489,-1.39381759281473,
131.984662666786));
#45772=CARTESIAN_POINT('Ctrl Pts',(0.818944543906922,-1.14429846421496,
132.011588370497));
#45773=CARTESIAN_POINT('Ctrl Pts',(1.2569512247398,-0.63258419209633,132.038514074207));
#45774=CARTESIAN_POINT('Ctrl Pts',(1.40695043465305,0.0240752216494901,
132.065439777918));
#45775=CARTESIAN_POINT('Ctrl Pts',(1.23457258791645,0.675218237060669,132.092365481628));
#45776=CARTESIAN_POINT('Ctrl Pts',(0.779314927371245,1.17164729590776,132.119291185338));
#45777=CARTESIAN_POINT('Ctrl Pts',(0.145491451718108,1.39961472504167,132.146216889049));
#45778=CARTESIAN_POINT('Ctrl Pts',(-0.52166873807337,1.30688594016532,132.173142592759));
#45779=CARTESIAN_POINT('Ctrl Pts',(-1.06929803713989,0.914708055599997,
132.200068296469));
#45780=CARTESIAN_POINT('Ctrl Pts',(-1.37191717032426,0.312941480414962,
132.22699400018));
#45781=CARTESIAN_POINT('Ctrl Pts',(-1.36018646259596,-0.360529924877197,
132.25391970389));
#45782=CARTESIAN_POINT('Ctrl Pts',(-1.03679379871711,-0.951392495179094,
132.2808454076));
#45783=CARTESIAN_POINT('Ctrl Pts',(-0.475838650423062,-1.32426076688091,
132.307771111311));
#45784=CARTESIAN_POINT('Ctrl Pts',(0.194146284383382,-1.39369894668277,
132.334696815021));
#45785=CARTESIAN_POINT('Ctrl Pts',(0.819646459479526,-1.14379618440796,
132.361622518732));
#45786=CARTESIAN_POINT('Ctrl Pts',(1.25733962810273,-0.631814008688681,
132.388548222442));
#45787=CARTESIAN_POINT('Ctrl Pts',(1.40693772775649,0.0249379681541858,
132.415473926152));
#45788=CARTESIAN_POINT('Ctrl Pts',(1.23416151766636,0.675972778138939,132.442399629863));
#45789=CARTESIAN_POINT('Ctrl Pts',(0.77860580590508,1.17212647107333,132.469325333573));
#45790=CARTESIAN_POINT('Ctrl Pts',(0.144644458248906,1.39969382955471,132.496251037283));
#45791=CARTESIAN_POINT('Ctrl Pts',(-0.522432283674648,1.30657564539846,
132.523176740994));
#45792=CARTESIAN_POINT('Ctrl Pts',(-1.06982053049778,0.914006906105429,
132.550102444704));
#45793=CARTESIAN_POINT('Ctrl Pts',(-1.27123964629225,0.512775424879935,
132.568052913844));
#45794=CARTESIAN_POINT('Ctrl Pts',(-1.31960187963311,0.300157166061732,
132.577028148414));
#45795=CARTESIAN_POINT('Ctrl Pts',(0.746857044345091,-1.04763739686597,
131.));
#45796=CARTESIAN_POINT('Ctrl Pts',(0.915655560497863,-0.927301523747248,
131.00897523457));
#45797=CARTESIAN_POINT('Ctrl Pts',(1.19383071914578,-0.603582305382327,
131.02692570371));
#45798=CARTESIAN_POINT('Ctrl Pts',(1.33763256702269,0.0204649803060436,
131.053851407421));
#45799=CARTESIAN_POINT('Ctrl Pts',(1.17488299294373,0.639781288322262,131.080777111131));
#45800=CARTESIAN_POINT('Ctrl Pts',(0.742945664266514,1.11253782599317,131.107702814841));
#45801=CARTESIAN_POINT('Ctrl Pts',(0.140763636876506,1.33036910873258,131.134628518552));
#45802=CARTESIAN_POINT('Ctrl Pts',(-0.49366903146045,1.24337802076997,131.161554222262));
#45803=CARTESIAN_POINT('Ctrl Pts',(-1.01498908290289,0.871488239228939,
131.188479925973));
#45804=CARTESIAN_POINT('Ctrl Pts',(-1.30374239775027,0.299914447706534,
131.215405629683));
#45805=CARTESIAN_POINT('Ctrl Pts',(-1.2937674765191,-0.340379470264034,
131.242331333393));
#45806=CARTESIAN_POINT('Ctrl Pts',(-0.98734923478118,-0.902681268882645,
131.269257037104));
#45807=CARTESIAN_POINT('Ctrl Pts',(-0.454698034476922,-1.2581501250631,
131.296182740814));
#45808=CARTESIAN_POINT('Ctrl Pts',(0.182138945505527,-1.32533672141841,
131.323108444524));
#45809=CARTESIAN_POINT('Ctrl Pts',(0.777242075774215,-1.08884655660415,
131.350034148235));
#45810=CARTESIAN_POINT('Ctrl Pts',(1.19425434657027,-0.602867023578126,
131.376959851945));
#45811=CARTESIAN_POINT('Ctrl Pts',(1.33762498699637,0.0212485044686996,
131.403885555655));
#45812=CARTESIAN_POINT('Ctrl Pts',(1.17450323342847,0.640495329295421,131.430811259366));
#45813=CARTESIAN_POINT('Ctrl Pts',(0.742265462285602,1.11298431999035,131.457736963076));
#45814=CARTESIAN_POINT('Ctrl Pts',(0.139951084671291,1.3304532338131,131.484662666786));
#45815=CARTESIAN_POINT('Ctrl Pts',(-0.494430534395506,1.24307303066064,
131.511588370497));
#45816=CARTESIAN_POINT('Ctrl Pts',(-1.01552240527922,0.870865292057418,
131.538514074207));
#45817=CARTESIAN_POINT('Ctrl Pts',(-1.30392582029322,0.299114639339331,
131.565439777918));
#45818=CARTESIAN_POINT('Ctrl Pts',(-1.29355839164082,-0.341172682937275,
131.592365481628));
#45819=CARTESIAN_POINT('Ctrl Pts',(-0.986795626701916,-0.903286501201301,
131.619291185338));
#45820=CARTESIAN_POINT('Ctrl Pts',(-0.453926623709776,-1.25842867593135,
131.646216889049));
#45821=CARTESIAN_POINT('Ctrl Pts',(0.182951394380693,-1.3252248486269,131.673142592759));
#45822=CARTESIAN_POINT('Ctrl Pts',(0.777909433892818,-1.08836989336796,
131.700068296469));
#45823=CARTESIAN_POINT('Ctrl Pts',(1.19462370043953,-0.602134807565142,
131.72699400018));
#45824=CARTESIAN_POINT('Ctrl Pts',(1.33761171253848,0.0220684982618089,
131.75391970389));
#45825=CARTESIAN_POINT('Ctrl Pts',(1.17411037251451,0.641215209809031,131.7808454076));
#45826=CARTESIAN_POINT('Ctrl Pts',(0.741583033376361,1.11343913921922,131.807771111311));
#45827=CARTESIAN_POINT('Ctrl Pts',(0.139135454071305,1.33053877717148,131.834696815021));
#45828=CARTESIAN_POINT('Ctrl Pts',(-0.495192479431881,1.24276969726887,
131.861622518732));
#45829=CARTESIAN_POINT('Ctrl Pts',(-1.01605607887236,0.870242584984128,
131.888548222442));
#45830=CARTESIAN_POINT('Ctrl Pts',(-1.3041089407751,0.298315240508559,131.915473926152));
#45831=CARTESIAN_POINT('Ctrl Pts',(-1.29334900026956,-0.341965605910532,
131.942399629863));
#45832=CARTESIAN_POINT('Ctrl Pts',(-0.986241701669955,-0.903891264481546,
131.969325333573));
#45833=CARTESIAN_POINT('Ctrl Pts',(-0.453155086833697,-1.25870670904991,
131.996251037283));
#45834=CARTESIAN_POINT('Ctrl Pts',(0.183763759504555,-1.32511244536446,
132.023176740994));
#45835=CARTESIAN_POINT('Ctrl Pts',(0.778576488622803,-1.08789280890088,
132.050102444704));
#45836=CARTESIAN_POINT('Ctrl Pts',(1.1949926014029,-0.601402357101034,132.077028148414));
#45837=CARTESIAN_POINT('Ctrl Pts',(1.3375979328864,0.02288848698503,132.103953852125));
#45838=CARTESIAN_POINT('Ctrl Pts',(1.17371706985718,0.641934851359759,132.130879555835));
#45839=CARTESIAN_POINT('Ctrl Pts',(0.740900326155663,1.11389354058136,132.157805259545));
#45840=CARTESIAN_POINT('Ctrl Pts',(0.138319773232647,1.3306238208134,132.184730963256));
#45841=CARTESIAN_POINT('Ctrl Pts',(-0.495954234429353,1.24246589576165,
132.211656666966));
#45842=CARTESIAN_POINT('Ctrl Pts',(-1.01658936156519,0.869619550362351,
132.238582370677));
#45843=CARTESIAN_POINT('Ctrl Pts',(-1.30429155563652,0.29751572408497,132.265508074387));
#45844=CARTESIAN_POINT('Ctrl Pts',(-1.29313908713286,-0.342758401704713,
132.292433778097));
#45845=CARTESIAN_POINT('Ctrl Pts',(-0.98568734749738,-0.904495711840062,
132.319359481808));
#45846=CARTESIAN_POINT('Ctrl Pts',(-0.452383239321647,-1.25898426892294,
132.346285185518));
#45847=CARTESIAN_POINT('Ctrl Pts',(0.184576273813673,-1.32499964763048,
132.373210889228));
#45848=CARTESIAN_POINT('Ctrl Pts',(0.779243804823753,-1.08741528786317,
132.400136592939));
#45849=CARTESIAN_POINT('Ctrl Pts',(1.19536185928334,-0.600670138176585,
132.427062296649));
#45850=CARTESIAN_POINT('Ctrl Pts',(1.33758585234813,0.0237087063139161,
132.453988000359));
#45851=CARTESIAN_POINT('Ctrl Pts',(1.17332626240353,0.642652199008768,132.48091370407));
#45852=CARTESIAN_POINT('Ctrl Pts',(0.740226159259698,1.11434909586972,132.50783940778));
#45853=CARTESIAN_POINT('Ctrl Pts',(0.137514530428304,1.33069902604488,132.53476511149));
#45854=CARTESIAN_POINT('Ctrl Pts',(-0.496680142743377,1.24217089628724,
132.561690815201));
#45855=CARTESIAN_POINT('Ctrl Pts',(-1.01708609977163,0.868952962477321,
132.588616518911));
#45856=CARTESIAN_POINT('Ctrl Pts',(-1.20857670689947,0.487499297388886,
132.606566988051));
#45857=CARTESIAN_POINT('Ctrl Pts',(-1.25455503119094,0.285361584158592,
132.615542222622));
#45858=CARTESIAN_POINT('Ctrl Pts',(0.855148668267253,0.961251009261909,
132.5));
#45859=CARTESIAN_POINT('Ctrl Pts',(0.817772472755866,0.999947679620164,
132.5));
#45860=CARTESIAN_POINT('Ctrl Pts',(0.778057507095388,1.03622562444653,132.5));
#45861=CARTESIAN_POINT('Ctrl Pts',(0.73623089071545,1.06985670395616,132.5));
#45862=CARTESIAN_POINT('Ctrl Pts',(0.730681434083883,1.07431879612054,132.5));
#45863=CARTESIAN_POINT('Ctrl Pts',(0.725094740290237,1.0787342570656,132.5));
#45864=CARTESIAN_POINT('Ctrl Pts',(0.719471281991385,1.08310251676537,132.5));
#45865=CARTESIAN_POINT('Ctrl Pts',(0.68847850560881,1.10717747008791,132.5));
#45866=CARTESIAN_POINT('Ctrl Pts',(0.656369876840734,1.12981958755506,132.5));
#45867=CARTESIAN_POINT('Ctrl Pts',(0.623260709674728,1.15099151444455,132.5));
#45868=CARTESIAN_POINT('Ctrl Pts',(0.612344806238366,1.15797177789632,132.5));
#45869=CARTESIAN_POINT('Ctrl Pts',(0.601320062392497,1.16479214312164,132.5));
#45870=CARTESIAN_POINT('Ctrl Pts',(0.590190382497418,1.1714509923087,132.5));
#45871=CARTESIAN_POINT('Ctrl Pts',(0.579798878378454,1.17766819346878,132.5));
#45872=CARTESIAN_POINT('Ctrl Pts',(0.569323560724368,1.18373997106925,132.5));
#45873=CARTESIAN_POINT('Ctrl Pts',(0.558770822371714,1.18966399771288,132.5));
#45874=CARTESIAN_POINT('Ctrl Pts',(0.511361729429498,1.21627820156729,132.5));
#45875=CARTESIAN_POINT('Ctrl Pts',(0.462375155234433,1.23992399549733,132.5));
#45876=CARTESIAN_POINT('Ctrl Pts',(0.412120795241606,1.26051510291273,132.5));
#45877=CARTESIAN_POINT('Ctrl Pts',(0.385984107461683,1.27122429004864,132.5));
#45878=CARTESIAN_POINT('Ctrl Pts',(0.35950388129632,1.28110658448462,132.5));
#45879=CARTESIAN_POINT('Ctrl Pts',(0.33272043457049,1.29014537761593,132.5));
#45880=CARTESIAN_POINT('Ctrl Pts',(0.317291476468849,1.29535229373617,132.5));
#45881=CARTESIAN_POINT('Ctrl Pts',(0.301761859550774,1.30027923535042,132.5));
#45882=CARTESIAN_POINT('Ctrl Pts',(0.286139050856096,1.30492251440297,132.5));
#45883=CARTESIAN_POINT('Ctrl Pts',(0.273481671713227,1.30868443356764,132.5));
#45884=CARTESIAN_POINT('Ctrl Pts',(0.260760780877808,1.31226060465732,132.5));
#45885=CARTESIAN_POINT('Ctrl Pts',(0.248002783150692,1.31564340253996,132.5));
#45886=CARTESIAN_POINT('Ctrl Pts',(0.21179126686695,1.32524492804826,132.5));
#45887=CARTESIAN_POINT('Ctrl Pts',(0.175243722368574,1.33330110003331,132.5));
#45888=CARTESIAN_POINT('Ctrl Pts',(0.138457680367238,1.33978673029291,132.5));
#45889=CARTESIAN_POINT('Ctrl Pts',(0.0840154582679713,1.34938526560242,
132.5));
#45890=CARTESIAN_POINT('Ctrl Pts',(0.0290514316829271,1.35554649398119,
132.5));
#45891=CARTESIAN_POINT('Ctrl Pts',(-0.0261190517268831,1.35834825553041,
132.5));
#45892=CARTESIAN_POINT('Ctrl Pts',(-0.0674969142842407,1.36044957669233,
132.5));
#45893=CARTESIAN_POINT('Ctrl Pts',(-0.108991568028323,1.36066014913089,
132.5));
#45894=CARTESIAN_POINT('Ctrl Pts',(-0.150474619481714,1.358993786071,132.5));
#45895=CARTESIAN_POINT('Ctrl Pts',(-0.171549637335457,1.35814720825168,
132.5));
#45896=CARTESIAN_POINT('Ctrl Pts',(-0.192621694545607,1.35681592531128,
132.5));
#45897=CARTESIAN_POINT('Ctrl Pts',(-0.213673988956076,1.35500012630149,
132.5));
#45898=CARTESIAN_POINT('Ctrl Pts',(-0.226286322656649,1.35391228938462,
132.5));
#45899=CARTESIAN_POINT('Ctrl Pts',(-0.238891562291373,1.35265053120959,
132.5));
#45900=CARTESIAN_POINT('Ctrl Pts',(-0.25148607234807,1.35121470346695,132.5));
#45901=CARTESIAN_POINT('Ctrl Pts',(-0.260958815768057,1.35013477040563,
132.5));
#45902=CARTESIAN_POINT('Ctrl Pts',(-0.270415802374623,1.34895746632245,
132.5));
#45903=CARTESIAN_POINT('Ctrl Pts',(-0.279855456160633,1.34768328952174,
132.5));
#45904=CARTESIAN_POINT('Ctrl Pts',(-0.335945831775187,1.34011213734059,
132.5));
#45905=CARTESIAN_POINT('Ctrl Pts',(-0.391423470349234,1.32912484896805,
132.5));
#45906=CARTESIAN_POINT('Ctrl Pts',(-0.445968675489026,1.31479535128022,
132.5));
#45907=CARTESIAN_POINT('Ctrl Pts',(-0.469964904553905,1.30849133412563,
132.5));
#45908=CARTESIAN_POINT('Ctrl Pts',(-0.493780806466491,1.30153978899266,
132.5));
#45909=CARTESIAN_POINT('Ctrl Pts',(-0.517389430066538,1.29394383943621,
132.5));
#45910=CARTESIAN_POINT('Ctrl Pts',(-0.57173464123408,1.27645855568328,132.5));
#45911=CARTESIAN_POINT('Ctrl Pts',(-0.624982569419363,1.25556235126801,
132.5));
#45912=CARTESIAN_POINT('Ctrl Pts',(-0.676874172622024,1.23144719124002,
132.5));
#45913=CARTESIAN_POINT('Ctrl Pts',(-0.697975522611471,1.22164093357219,
132.5));
#45914=CARTESIAN_POINT('Ctrl Pts',(-0.718852426177283,1.21130177645272,
132.5));
#45915=CARTESIAN_POINT('Ctrl Pts',(-0.739486538730255,1.20044020333604,
132.5));
#45916=CARTESIAN_POINT('Ctrl Pts',(-0.748608547965024,1.19563847658282,
132.5));
#45917=CARTESIAN_POINT('Ctrl Pts',(-0.757684868562274,1.19073364697938,
132.5));
#45918=CARTESIAN_POINT('Ctrl Pts',(-0.766708209897055,1.18572968739322,
132.5));
#45919=CARTESIAN_POINT('Ctrl Pts',(-0.816798485324484,1.15795176072512,
132.5));
#45920=CARTESIAN_POINT('Ctrl Pts',(-0.865077227104213,1.12722452484418,
132.5));
#45921=CARTESIAN_POINT('Ctrl Pts',(-0.911304538955749,1.09377557298447,
132.5));
#45922=CARTESIAN_POINT('Ctrl Pts',(-0.958041120987901,1.05995812568187,
132.5));
#45923=CARTESIAN_POINT('Ctrl Pts',(-1.00268180188713,1.02335824079455,132.5));
#45924=CARTESIAN_POINT('Ctrl Pts',(-1.04496242001946,0.984161078201646,
132.5));
#45925=CARTESIAN_POINT('Ctrl Pts',(-1.06200634880544,0.968360134947809,
132.5));
#45926=CARTESIAN_POINT('Ctrl Pts',(-1.07866649907554,0.95213660337011,132.5));
#45927=CARTESIAN_POINT('Ctrl Pts',(-1.09492426754628,0.935500592349208,
132.5));
#45928=CARTESIAN_POINT('Ctrl Pts',(-1.11554174922657,0.914403437898156,
132.5));
#45929=CARTESIAN_POINT('Ctrl Pts',(-1.13551220287225,0.892642983461476,
132.5));
#45930=CARTESIAN_POINT('Ctrl Pts',(-1.15481600835651,0.870254551841039,
132.5));
#45931=CARTESIAN_POINT('Ctrl Pts',(-1.16444119992803,0.859091315477714,
132.5));
#45932=CARTESIAN_POINT('Ctrl Pts',(-1.17390060984583,0.84777191375158,132.5));
#45933=CARTESIAN_POINT('Ctrl Pts',(-1.18319154863334,0.836300512267484,
132.5));
#45934=CARTESIAN_POINT('Ctrl Pts',(-1.18967862373224,0.828291004873353,
132.5));
#45935=CARTESIAN_POINT('Ctrl Pts',(-1.19608091416041,0.820210558598525,
132.5));
#45936=CARTESIAN_POINT('Ctrl Pts',(-1.20239194526469,0.812068424359708,
132.5));
#45937=CARTESIAN_POINT('Ctrl Pts',(-1.23816283253369,0.765918855268116,
132.5));
#45938=CARTESIAN_POINT('Ctrl Pts',(-1.27106156977561,0.717720815582551,
132.5));
#45939=CARTESIAN_POINT('Ctrl Pts',(-1.30098385596562,0.667789887343701,
132.5));
#45940=CARTESIAN_POINT('Ctrl Pts',(-1.33267614741923,0.614905374434283,
132.5));
#45941=CARTESIAN_POINT('Ctrl Pts',(-1.36103053192321,0.560076290633097,
132.5));
#45942=CARTESIAN_POINT('Ctrl Pts',(-1.38588025440444,0.503631907907152,
132.5));
#45943=CARTESIAN_POINT('Ctrl Pts',(-1.40936682016066,0.450283839031791,
132.5));
#45944=CARTESIAN_POINT('Ctrl Pts',(-1.42972289617106,0.395491656254383,
132.5));
#45945=CARTESIAN_POINT('Ctrl Pts',(-1.44676228694776,0.339508156752185,
132.5));
#45946=CARTESIAN_POINT('Ctrl Pts',(-1.44775125061185,0.336258882906532,
132.5));
#45947=CARTESIAN_POINT('Ctrl Pts',(-1.44872902769048,0.33300559132195,132.5));
#45948=CARTESIAN_POINT('Ctrl Pts',(-1.44969557651745,0.32974832986801,132.5));
#45949=CARTESIAN_POINT('Ctrl Pts',(0.644080091014819,1.33993887967342,131.));
#45950=CARTESIAN_POINT('Ctrl Pts',(0.69545855375229,1.31106406966807,131.));
#45951=CARTESIAN_POINT('Ctrl Pts',(0.74501305727242,1.27920888146368,131.));
#45952=CARTESIAN_POINT('Ctrl Pts',(0.79244836341944,1.2444798284805,131.));
#45953=CARTESIAN_POINT('Ctrl Pts',(0.801096314078014,1.23814836019216,131.));
#45954=CARTESIAN_POINT('Ctrl Pts',(0.809673740649968,1.23172126484837,131.));
#45955=CARTESIAN_POINT('Ctrl Pts',(0.818178728015053,1.22519904766394,131.));
#45956=CARTESIAN_POINT('Ctrl Pts',(0.849870741953171,1.20089540216238,131.));
#45957=CARTESIAN_POINT('Ctrl Pts',(0.880557609427367,1.17527144874649,131.));
#45958=CARTESIAN_POINT('Ctrl Pts',(0.910170030271529,1.14840188938563,131.));
#45959=CARTESIAN_POINT('Ctrl Pts',(0.924142438892699,1.1357236803045,131.));
#45960=CARTESIAN_POINT('Ctrl Pts',(0.937875509062744,1.12276806491419,131.));
#45961=CARTESIAN_POINT('Ctrl Pts',(0.951361230019935,1.10954246813862,131.));
#45962=CARTESIAN_POINT('Ctrl Pts',(0.960549382748327,1.10053154440056,131.));
#45963=CARTESIAN_POINT('Ctrl Pts',(0.969616382834828,1.09140144700476,131.));
#45964=CARTESIAN_POINT('Ctrl Pts',(0.978557707856144,1.08215751935785,131.));
#45965=CARTESIAN_POINT('Ctrl Pts',(1.01915721296604,1.04018399900805,131.));
#45966=CARTESIAN_POINT('Ctrl Pts',(1.05718615879812,0.995849105860942,131.));
#45967=CARTESIAN_POINT('Ctrl Pts',(1.09243705884413,0.949397585827403,131.));
#45968=CARTESIAN_POINT('Ctrl Pts',(1.10966817281199,0.92669145819283,131.));
#45969=CARTESIAN_POINT('Ctrl Pts',(1.12623485703778,0.903479138792705,131.));
#45970=CARTESIAN_POINT('Ctrl Pts',(1.14210882027374,0.879787145895407,131.));
#45971=CARTESIAN_POINT('Ctrl Pts',(1.15509929664831,0.860398775806344,131.));
#45972=CARTESIAN_POINT('Ctrl Pts',(1.16762581229777,0.840689140294072,131.));
#45973=CARTESIAN_POINT('Ctrl Pts',(1.1796713745992,0.820672327962755,131.));
#45974=CARTESIAN_POINT('Ctrl Pts',(1.18580410439404,0.810481213732452,131.));
#45975=CARTESIAN_POINT('Ctrl Pts',(1.19181264491176,0.800209353684452,131.));
#45976=CARTESIAN_POINT('Ctrl Pts',(1.19768623361316,0.789874026042805,131.));
#45977=CARTESIAN_POINT('Ctrl Pts',(1.21764656797304,0.754751274700468,131.));
#45978=CARTESIAN_POINT('Ctrl Pts',(1.2360737454091,0.718856382057069,131.));
#45979=CARTESIAN_POINT('Ctrl Pts',(1.25290111099389,0.682270801499543,131.));
#45980=CARTESIAN_POINT('Ctrl Pts',(1.27683978739331,0.630224010845455,131.));
#45981=CARTESIAN_POINT('Ctrl Pts',(1.29754304910658,0.576779540065319,131.));
#45982=CARTESIAN_POINT('Ctrl Pts',(1.31495193836166,0.522251731680102,131.));
#45983=CARTESIAN_POINT('Ctrl Pts',(1.3278134384389,0.481967173516586,131.));
#45984=CARTESIAN_POINT('Ctrl Pts',(1.3388758149635,0.441090831843476,131.));
#45985=CARTESIAN_POINT('Ctrl Pts',(1.34809711264878,0.399747850113526,131.));
#45986=CARTESIAN_POINT('Ctrl Pts',(1.3522739374108,0.381021376278836,131.));
#45987=CARTESIAN_POINT('Ctrl Pts',(1.35607281945074,0.362199171744182,131.));
#45988=CARTESIAN_POINT('Ctrl Pts',(1.35948878751085,0.343293002470523,131.));
#45989=CARTESIAN_POINT('Ctrl Pts',(1.36178540468056,0.330582042589365,131.));
#45990=CARTESIAN_POINT('Ctrl Pts',(1.36390892640178,0.31783313200029,131.));
#45991=CARTESIAN_POINT('Ctrl Pts',(1.36585766900664,0.305049889819707,131.));
#45992=CARTESIAN_POINT('Ctrl Pts',(1.36749890793905,0.294283791363784,131.));
#45993=CARTESIAN_POINT('Ctrl Pts',(1.36901622844932,0.283492059509838,131.));
#45994=CARTESIAN_POINT('Ctrl Pts',(1.37040659854361,0.272694555744875,131.));
#45995=CARTESIAN_POINT('Ctrl Pts',(1.37758020654124,0.216984885578319,131.));
#45996=CARTESIAN_POINT('Ctrl Pts',(1.38139594905319,0.161015108050636,131.));
#45997=CARTESIAN_POINT('Ctrl Pts',(1.38179530614646,0.105081015157366,131.));
#45998=CARTESIAN_POINT('Ctrl Pts',(1.38199532044291,0.077066943476098,131.));
#45999=CARTESIAN_POINT('Ctrl Pts',(1.38133755560142,0.0490617639963321,
131.));
#46000=CARTESIAN_POINT('Ctrl Pts',(1.37980973540542,0.0211029507209763,
131.));
#46001=CARTESIAN_POINT('Ctrl Pts',(1.37682437540304,-0.0335285583302587,
131.));
#46002=CARTESIAN_POINT('Ctrl Pts',(1.37051962444526,-0.0879843276874055,
131.));
#46003=CARTESIAN_POINT('Ctrl Pts',(1.36095581982918,-0.141970240438976,
131.));
#46004=CARTESIAN_POINT('Ctrl Pts',(1.35717999267375,-0.16328408817649,131.));
#46005=CARTESIAN_POINT('Ctrl Pts',(1.35289570340238,-0.184524487242908,
131.));
#46006=CARTESIAN_POINT('Ctrl Pts',(1.34810488396129,-0.205672316005588,
131.));
#46007=CARTESIAN_POINT('Ctrl Pts',(1.34573474475713,-0.216134680252416,
131.));
#46008=CARTESIAN_POINT('Ctrl Pts',(1.34324061587303,-0.226574376939408,
131.));
#46009=CARTESIAN_POINT('Ctrl Pts',(1.34062264574658,-0.236989022514862,
131.));
#46010=CARTESIAN_POINT('Ctrl Pts',(1.33809205801851,-0.247056048879768,
131.));
#46011=CARTESIAN_POINT('Ctrl Pts',(1.33544770532017,-0.257091762818921,
131.));
#46012=CARTESIAN_POINT('Ctrl Pts',(1.33269167226224,-0.267089239813752,
131.));
#46013=CARTESIAN_POINT('Ctrl Pts',(1.31803859533809,-0.320243101314323,
131.));
#46014=CARTESIAN_POINT('Ctrl Pts',(1.30022114977825,-0.37236300147042,131.));
#46015=CARTESIAN_POINT('Ctrl Pts',(1.27933280126981,-0.423158242313197,
131.));
#46016=CARTESIAN_POINT('Ctrl Pts',(1.2587042121418,-0.473321813290589,131.));
#46017=CARTESIAN_POINT('Ctrl Pts',(1.23508013373137,-0.522194372177886,
131.));
#46018=CARTESIAN_POINT('Ctrl Pts',(1.20850705635476,-0.569470695394981,
131.));
#46019=CARTESIAN_POINT('Ctrl Pts',(1.20244994149213,-0.580246945204162,
131.));
#46020=CARTESIAN_POINT('Ctrl Pts',(1.19623944020916,-0.590940122396141,
131.));
#46021=CARTESIAN_POINT('Ctrl Pts',(1.18987582062145,-0.601546350856353,
131.));
#46022=CARTESIAN_POINT('Ctrl Pts',(1.17627259476364,-0.624218812535633,
131.));
#46023=CARTESIAN_POINT('Ctrl Pts',(1.16196977799215,-0.646494107742248,
131.));
#46024=CARTESIAN_POINT('Ctrl Pts',(1.14698856130615,-0.668343080492641,
131.));
#46025=CARTESIAN_POINT('Ctrl Pts',(1.13947209480414,-0.679305279039234,
131.));
#46026=CARTESIAN_POINT('Ctrl Pts',(1.13178483051549,-0.690160123296984,
131.));
#46027=CARTESIAN_POINT('Ctrl Pts',(1.12392930861312,-0.700903697400656,
131.));
#46028=CARTESIAN_POINT('Ctrl Pts',(1.11818104819913,-0.708765283491613,
131.));
#46029=CARTESIAN_POINT('Ctrl Pts',(1.11234308420749,-0.716566584269759,
131.));
#46030=CARTESIAN_POINT('Ctrl Pts',(1.10642468674068,-0.724295734963858,
131.));
#46031=CARTESIAN_POINT('Ctrl Pts',(1.07360868842271,-0.767151896213436,
131.));
#46032=CARTESIAN_POINT('Ctrl Pts',(1.03826013572302,-0.807879761409639,
131.));
#46033=CARTESIAN_POINT('Ctrl Pts',(1.00060431004052,-0.846274730734576,
131.));
#46034=CARTESIAN_POINT('Ctrl Pts',(0.962725613573854,-0.884896945559157,
131.));
#46035=CARTESIAN_POINT('Ctrl Pts',(0.92251141476043,-0.921159328591376,
131.));
#46036=CARTESIAN_POINT('Ctrl Pts',(0.88015838080179,-0.954811648572381,
131.));
#46037=CARTESIAN_POINT('Ctrl Pts',(0.83780534684315,-0.988463968553386,
131.));
#46038=CARTESIAN_POINT('Ctrl Pts',(0.793312631206348,-1.01950695396809,
131.));
#46039=CARTESIAN_POINT('Ctrl Pts',(0.746857044345091,-1.04763739686597,
131.));
#46040=CARTESIAN_POINT('Origin',(0.,0.,131.75));
#46041=CARTESIAN_POINT('Origin',(0.,0.,132.5));
#46042=CARTESIAN_POINT('Origin',(2.55,0.,111.5));
#46043=CARTESIAN_POINT('',(-2.55,-3.12284933782575E-16,111.5));
#46044=CARTESIAN_POINT('Origin',(0.,0.,111.5));
#46045=CARTESIAN_POINT('Origin',(0.,0.,111.55));
#46046=CARTESIAN_POINT('',(-2.65,-3.24531401774049E-16,111.6));
#46047=CARTESIAN_POINT('Origin',(0.,0.,111.6));
#46048=CARTESIAN_POINT('',(-2.6,-3.18408167778312E-16,111.55));
#46049=CARTESIAN_POINT('Origin',(0.,0.,121.225));
#46050=CARTESIAN_POINT('',(-2.65,-3.24531401774049E-16,130.85));
#46051=CARTESIAN_POINT('Origin',(0.,0.,130.85));
#46052=CARTESIAN_POINT('',(-2.65,-3.24531401774049E-16,121.225));
#46053=CARTESIAN_POINT('Origin',(0.,0.,130.925));
#46054=CARTESIAN_POINT('',(-2.50000000000001,-3.06161699786839E-16,131.));
#46055=CARTESIAN_POINT('Origin',(0.,0.,131.));
#46056=CARTESIAN_POINT('',(-2.575,-3.15346550780443E-16,130.925));
#46057=CARTESIAN_POINT('Origin',(1.5,0.,131.));
#46058=CARTESIAN_POINT('Origin',(2.15,0.,132.5));
#46059=CARTESIAN_POINT('',(-2.14999999999999,-2.6329906181668E-16,132.5));
#46060=CARTESIAN_POINT('Origin',(0.,0.,132.5));
#46061=CARTESIAN_POINT('Origin',(0.,0.,132.55));
#46062=CARTESIAN_POINT('Origin',(0.,0.,132.6));
#46063=CARTESIAN_POINT('',(-2.2,-2.69422295812418E-16,132.55));
#46064=CARTESIAN_POINT('Origin',(0.,0.,133.225));
#46065=CARTESIAN_POINT('Origin',(0.,0.,134.));
#71457=UNCERTAINTY_MEASURE_WITH_UNIT(LENGTH_MEASURE(0.001),#71493,
'DISTANCE_ACCURACY_VALUE',
'Maximum model space distance between geometric entities at asserted c
onnectivities');
#71471=UNCERTAINTY_MEASURE_WITH_UNIT(LENGTH_MEASURE(0.001),#71493,
'DISTANCE_ACCURACY_VALUE',
'Maximum model space distance between geometric entities at asserted c
onnectivities');
#71478=(
GEOMETRIC_REPRESENTATION_CONTEXT(3)
GLOBAL_UNCERTAINTY_ASSIGNED_CONTEXT((#71457))
GLOBAL_UNIT_ASSIGNED_CONTEXT((#71493,#71495,#71496))
REPRESENTATION_CONTEXT('','3D')
);
#71492=(
GEOMETRIC_REPRESENTATION_CONTEXT(3)
GLOBAL_UNCERTAINTY_ASSIGNED_CONTEXT((#71471))
GLOBAL_UNIT_ASSIGNED_CONTEXT((#71493,#71495,#71496))
REPRESENTATION_CONTEXT('','3D')
);
#71493=(
LENGTH_UNIT()
NAMED_UNIT(*)
SI_UNIT(.CENTI.,.METRE.)
);
#71495=(
NAMED_UNIT(*)
PLANE_ANGLE_UNIT()
SI_UNIT($,.RADIAN.)
);
#71496=(
NAMED_UNIT(*)
SI_UNIT($,.STERADIAN.)
SOLID_ANGLE_UNIT()
);
#71503=SHAPE_DEFINITION_REPRESENTATION(#71523,#71608);
#71523=PRODUCT_DEFINITION_SHAPE('',$,#71629);
#71608=SHAPE_REPRESENTATION('',(#29535),#71478);
#71622=PRODUCT_DEFINITION_CONTEXT('part definition',#71684,'design');
#71629=PRODUCT_DEFINITION('2026-10-19-03-22-19-429',
'10_Jack_Ram_D53_Extension_Screw_M30',#71649,#71622);
#71649=PRODUCT_DEFINITION_FORMATION('',$,#71692);
#71684=APPLICATION_CONTEXT(
'Core Data for Automotive Mechanical Design Process');
#71685=PRODUCT_CONTEXT('part definition',#71684,'mechanical');
#71692=PRODUCT('2026-10-19-03-22-19-429',
'10_Jack_Ram_D53_Extension_Screw_M30',$,(#71685));
#71888=COLOUR_RGB('Black',0.12,0.14,0.17);
#71889=FILL_AREA_STYLE_COLOUR('',#71888);
#71890=FILL_AREA_STYLE('',(#71889));
#71891=SURFACE_STYLE_FILL_AREA(#71890);
#71892=SURFACE_SIDE_STYLE('',(#71891));
#71893=SURFACE_STYLE_USAGE(.BOTH.,#71892);
#71894=PRESENTATION_STYLE_ASSIGNMENT((#71893));
ENDSEC;
END-ISO-10303-21;
